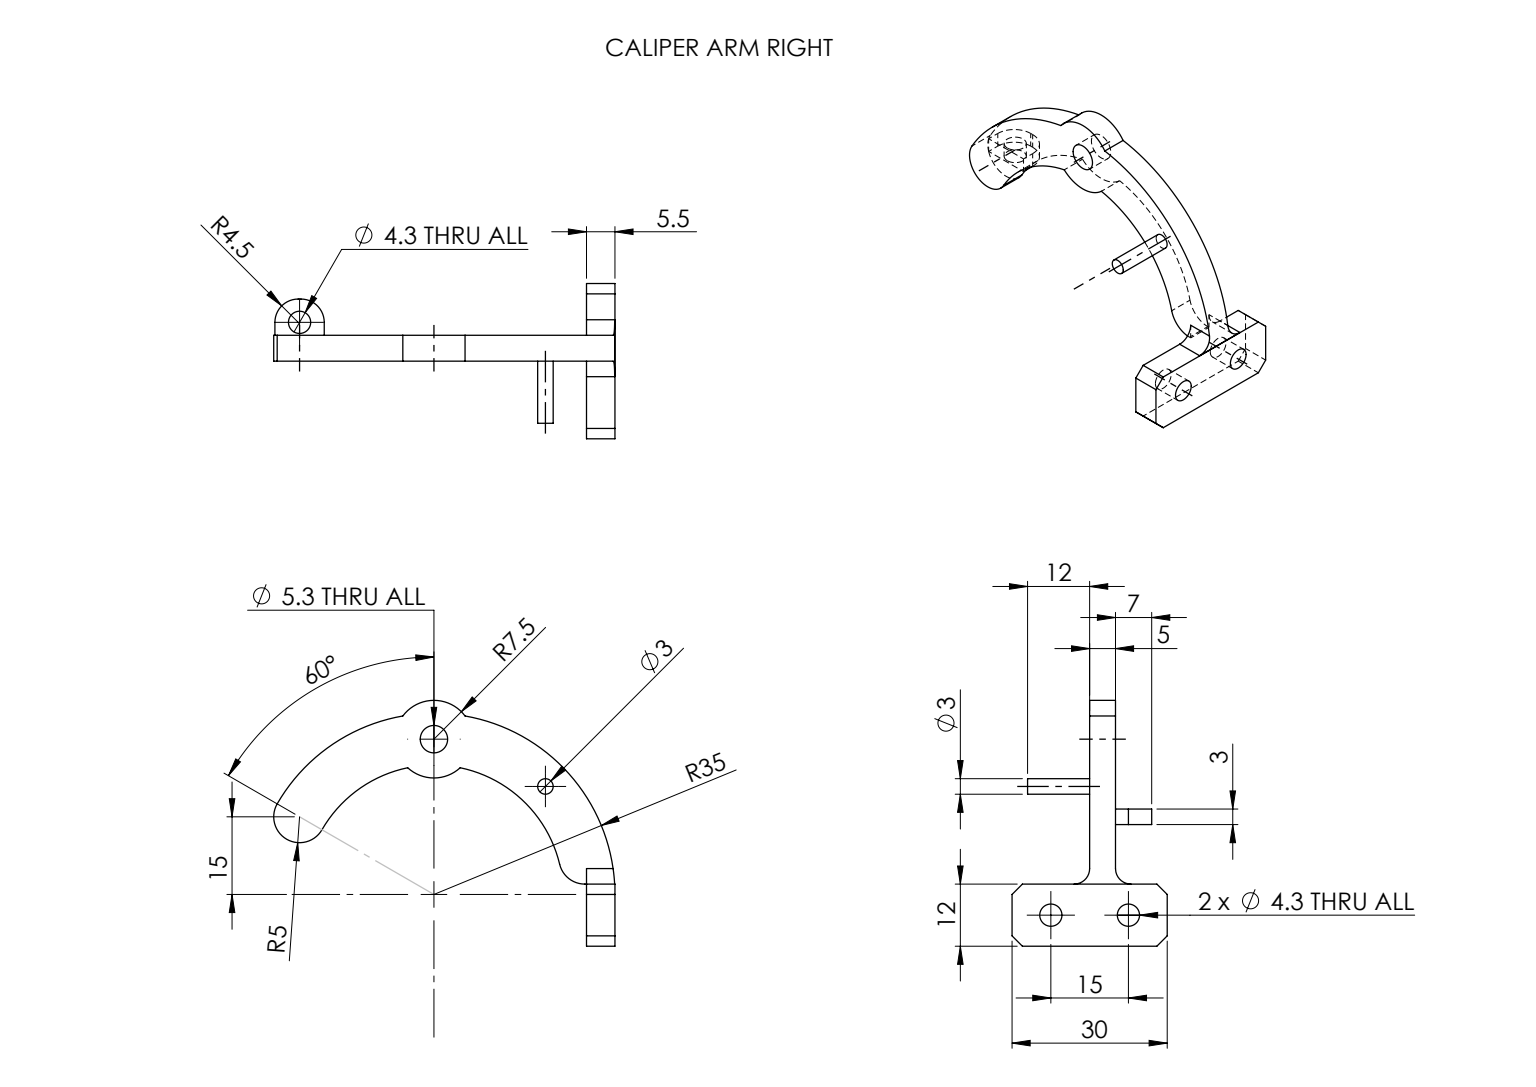
ISO-10303-21;
HEADER;
FILE_DESCRIPTION (('STEP AP214'),
    '1' );
FILE_NAME ('caliper arm right.step',
    '2026-10-08T05:45:04',
    ( '' ),
    ( '' ),
    'SwSTEP 2.0',
    'SolidWorks 2026',
    '' );
FILE_SCHEMA (( 'AUTOMOTIVE_DESIGN' ));
ENDSEC;

DATA;
#18=UNCERTAINTY_MEASURE_WITH_UNIT (LENGTH_MEASURE( 1.000000000000000082E-05 ), #5479, 'distance_accuracy_value', 'NONE');
#20=EDGE_CURVE ( 'NONE', #10326, #5059, #2301, .T. ) ;
#29=DIRECTION ( 'NONE',  ( 6.098637220230963674E-17, -1.000000000000000000, 0.000000000000000000 ) ) ;
#33=ADVANCED_FACE ( 'NONE', ( #727 ), #6680, .T. ) ;
#37=ORIENTED_EDGE ( 'NONE', *, *, #2342, .T. ) ;
#39=CARTESIAN_POINT ( 'NONE',  ( 34.64101615137754209, 5.000000000000000888, 2.500000000000000000 ) ) ;
#46=CARTESIAN_POINT ( 'NONE',  ( 29.49999999999999289, -3.999999999999993339, 12.14999999999999503 ) ) ;
#49=ADVANCED_FACE ( 'NONE', ( #5029 ), #6019, .T. ) ;
#84=LINE ( 'NONE', #3373, #8593 ) ;
#89=DIRECTION ( 'NONE',  ( 1.156482317317871478E-16, -0.000000000000000000, -1.000000000000000000 ) ) ;
#107=EDGE_CURVE ( 'NONE', #8667, #6915, #8632, .T. ) ;
#117=ORIENTED_EDGE ( 'NONE', *, *, #2558, .T. ) ;
#119=FILL_AREA_STYLE_COLOUR ( '', #3145 ) ;
#126=DIRECTION ( 'NONE',  ( -4.029251166000348040E-16, -0.7071067811865463515, 0.7071067811865486830 ) ) ;
#129=EDGE_CURVE ( 'NONE', #9236, #8327, #4531, .T. ) ;
#132=CARTESIAN_POINT ( 'NONE',  ( -30.75045812061784289, 13.49999999999941913, -5.000000000000000000 ) ) ;
#143=VERTEX_POINT ( 'NONE', #4423 ) ;
#157=DIRECTION ( 'NONE',  ( -1.000000000000000000, 0.000000000000000000, 0.000000000000000000 ) ) ;
#162=CARTESIAN_POINT ( 'NONE',  ( -6.015568632492056977, 34.47916666666665009, 0.000000000000000000 ) ) ;
#167=ADVANCED_FACE ( 'NONE', ( #9404 ), #2582, .F. ) ;
#169=DIRECTION ( 'NONE',  ( -1.000000000000000000, 0.000000000000000000, 0.000000000000000000 ) ) ;
#180=CARTESIAN_POINT ( 'NONE',  ( 0.000000000000000000, 0.000000000000000000, -2.500000000000000000 ) ) ;
#188=DIRECTION ( 'NONE',  ( 1.000000000000000000, 6.098637220230964906E-17, 0.000000000000000000 ) ) ;
#191=LINE ( 'NONE', #5261, #9329 ) ;
#195=CIRCLE ( 'NONE', #3924, 7.500000000000000000 ) ;
#203=EDGE_LOOP ( 'NONE', ( #3359, #5772 ) ) ;
#204=ORIENTED_EDGE ( 'NONE', *, *, #3358, .T. ) ;
#224=PRESENTATION_STYLE_ASSIGNMENT (( #9345 ) ) ;
#231=CARTESIAN_POINT ( 'NONE',  ( 34.99999999999999289, 2.000000000000002220, -12.49999999999999822 ) ) ;
#234=VERTEX_POINT ( 'NONE', #10467 ) ;
#236=EDGE_CURVE ( 'NONE', #3617, #2973, #5354, .T. ) ;
#238=DIRECTION ( 'NONE',  ( 0.000000000000000000, 0.000000000000000000, 1.000000000000000000 ) ) ;
#241=DIRECTION ( 'NONE',  ( 4.312387734421983755E-17, -0.7071067811865462405, -0.7071067811865489050 ) ) ;
#242=EDGE_CURVE ( 'NONE', #1228, #6486, #8792, .T. ) ;
#253=EDGE_CURVE ( 'NONE', #7504, #6853, #3627, .T. ) ;
#254=CARTESIAN_POINT ( 'NONE',  ( -25.98076211353324894, 16.50000000000026290, -7.149999999999990585 ) ) ;
#267=VECTOR ( 'NONE', #7158, 1000.000000000000000 ) ;
#268=DIRECTION ( 'NONE',  ( 0.000000000000000000, 0.000000000000000000, 1.000000000000000000 ) ) ;
#269=VECTOR ( 'NONE', #6345, 1000.000000000000000 ) ;
#270=VECTOR ( 'NONE', #9575, 1000.000000000000000 ) ;
#286=AXIS2_PLACEMENT_3D ( 'NONE', #4193, #3362, #6741 ) ;
#308=AXIS2_PLACEMENT_3D ( 'NONE', #6956, #4296, #9565 ) ;
#317=EDGE_LOOP ( 'NONE', ( #5235, #5389 ) ) ;
#326=CIRCLE ( 'NONE', #6705, 2.649999999999991029 ) ;
#331=CARTESIAN_POINT ( 'NONE',  ( -21.21106610644865498, 16.50000000000026290, -9.500000000000000000 ) ) ;
#334=ORIENTED_EDGE ( 'NONE', *, *, #9479, .T. ) ;
#342=ORIENTED_EDGE ( 'NONE', *, *, #1250, .F. ) ;
#346=CARTESIAN_POINT ( 'NONE',  ( -25.98076211353324894, 14.99999999999984190, -2.500000000000000000 ) ) ;
#348=CARTESIAN_POINT ( 'NONE',  ( -21.21106610644865498, 13.49999999999941913, -5.000000000000000000 ) ) ;
#350=CARTESIAN_POINT ( 'NONE',  ( 20.05579831881754060, 20.86490736922957367, 14.50000000000000000 ) ) ;
#360=ADVANCED_FACE ( 'NONE', ( #8018 ), #2971, .F. ) ;
#361=CARTESIAN_POINT ( 'NONE',  ( 34.99999999999999289, -3.999999999999993339, 10.00000000000000533 ) ) ;
#364=DIRECTION ( 'NONE',  ( 6.098637220230964906E-17, -1.000000000000000000, 0.000000000000000000 ) ) ;
#374=CYLINDRICAL_SURFACE ( 'NONE', #7364, 7.500000000000000000 ) ;
#398=DIRECTION ( 'NONE',  ( -4.312387734421998546E-17, 0.7071067811865489050, -0.7071067811865462405 ) ) ;
#420=VECTOR ( 'NONE', #4987, 1000.000000000000000 ) ;
#421=EDGE_CURVE ( 'NONE', #10496, #6333, #10386, .T. ) ;
#429=EDGE_CURVE ( 'NONE', #7102, #2953, #8173, .T. ) ;
#446=AXIS2_PLACEMENT_3D ( 'NONE', #473, #2203, #364 ) ;
#447=DIRECTION ( 'NONE',  ( 0.000000000000000000, 0.000000000000000000, -1.000000000000000000 ) ) ;
#448=FACE_BOUND ( 'NONE', #1109, .T. ) ;
#450=ORIENTED_EDGE ( 'NONE', *, *, #5486, .T. ) ;
#457=EDGE_CURVE ( 'NONE', #3885, #9988, #8075, .T. ) ;
#468=CARTESIAN_POINT ( 'NONE',  ( -25.71106610644865498, 13.49999999999941913, -5.000000000000000000 ) ) ;
#473=CARTESIAN_POINT ( 'NONE',  ( -3.049318610115482207E-16, 5.000000000000000000, -5.500000000000000000 ) ) ;
#480=DIRECTION ( 'NONE',  ( 0.000000000000000000, 0.000000000000000000, 1.000000000000000000 ) ) ;
#495=ORIENTED_EDGE ( 'NONE', *, *, #3771, .F. ) ;
#510=DIRECTION ( 'NONE',  ( 1.000000000000000000, 0.000000000000000000, 0.000000000000000000 ) ) ;
#515=UNCERTAINTY_MEASURE_WITH_UNIT (LENGTH_MEASURE( 1.000000000000000082E-05 ), #7040, 'distance_accuracy_value', 'NONE');
#517=DIRECTION ( 'NONE',  ( 0.000000000000000000, 0.000000000000000000, 1.000000000000000000 ) ) ;
#519=CARTESIAN_POINT ( 'NONE',  ( -25.98076211353324894, 13.49999999999941913, -7.149999999999990585 ) ) ;
#528=CARTESIAN_POINT ( 'NONE',  ( 0.000000000000000000, 0.000000000000000000, -2.500000000000000000 ) ) ;
#545=ADVANCED_FACE ( 'NONE', ( #10947 ), #7561, .T. ) ;
#551=ORIENTED_EDGE ( 'NONE', *, *, #3434, .F. ) ;
#555=EDGE_CURVE ( 'NONE', #6915, #590, #2328, .T. ) ;
#563=EDGE_LOOP ( 'NONE', ( #7565, #8832, #8917, #5557 ) ) ;
#564=DIRECTION ( 'NONE',  ( -1.000000000000000000, 0.000000000000000000, 0.000000000000000000 ) ) ;
#568=AXIS2_PLACEMENT_3D ( 'NONE', #528, #9502, #169 ) ;
#573=EDGE_CURVE ( 'NONE', #652, #6838, #3756, .T. ) ;
#575=FACE_OUTER_BOUND ( 'NONE', #2113, .T. ) ;
#577=ORIENTED_EDGE ( 'NONE', *, *, #9425, .T. ) ;
#589=ADVANCED_FACE ( 'NONE', ( #5232 ), #5948, .F. ) ;
#590=VERTEX_POINT ( 'NONE', #5013 ) ;
#599=AXIS2_PLACEMENT_3D ( 'NONE', #2316, #6635, #3978 ) ;
#603=EDGE_CURVE ( 'NONE', #9227, #143, #8788, .T. ) ;
#609=VERTEX_POINT ( 'NONE', #8450 ) ;
#616=DIRECTION ( 'NONE',  ( 1.000000000000000000, -0.000000000000000000, -0.000000000000000000 ) ) ;
#618=CARTESIAN_POINT ( 'NONE',  ( 34.99999999999999289, 2.000000000000002220, 15.50000000000000533 ) ) ;
#622=DIRECTION ( 'NONE',  ( -6.098637220230964906E-17, 1.000000000000000000, 0.000000000000000000 ) ) ;
#624=EDGE_CURVE ( 'NONE', #7008, #1215, #7866, .T. ) ;
#628=AXIS2_PLACEMENT_3D ( 'NONE', #1690, #8407, #6856 ) ;
#631=CARTESIAN_POINT ( 'NONE',  ( 29.49999999999999289, 2.000000000000001776, 17.50000000000000000 ) ) ;
#652=VERTEX_POINT ( 'NONE', #7794 ) ;
#659=CARTESIAN_POINT ( 'NONE',  ( 0.000000000000000000, 30.00000000000000000, -2.499999999999998668 ) ) ;
#663=AXIS2_PLACEMENT_3D ( 'NONE', #9560, #2957, #1054 ) ;
#666=PRODUCT_DEFINITION_CONTEXT ( 'detailed design', #7209, 'design' ) ;
#667=ORIENTED_EDGE ( 'NONE', *, *, #6516, .T. ) ;
#670=VERTEX_POINT ( 'NONE', #1318 ) ;
#672=VECTOR ( 'NONE', #10406, 1000.000000000000000 ) ;
#674=VECTOR ( 'NONE', #5477, 1000.000000000000000 ) ;
#680=DIRECTION ( 'NONE',  ( -0.000000000000000000, -0.000000000000000000, -1.000000000000000000 ) ) ;
#690=EDGE_LOOP ( 'NONE', ( #9028, #6042, #6525, #4019, #7005, #10810 ) ) ;
#691=DIRECTION ( 'NONE',  ( -1.000000000000000000, -6.098637220230964906E-17, -0.000000000000000000 ) ) ;
#727=FACE_OUTER_BOUND ( 'NONE', #7562, .T. ) ;
#730=EDGE_LOOP ( 'NONE', ( #3773, #3925, #4540, #10930 ) ) ;
#752=DIRECTION ( 'NONE',  ( 1.000000000000000000, -0.000000000000000000, -0.000000000000000000 ) ) ;
#753=EDGE_LOOP ( 'NONE', ( #8453, #4556, #9444, #8263 ) ) ;
#761=EDGE_CURVE ( 'NONE', #652, #9304, #1958, .T. ) ;
#763=LINE ( 'NONE', #4112, #7788 ) ;
#768=ORIENTED_EDGE ( 'NONE', *, *, #5709, .F. ) ;
#777=LINE ( 'NONE', #3237, #3403 ) ;
#780=AXIS2_PLACEMENT_3D ( 'NONE', #1700, #10147, #4202 ) ;
#785=PLANE ( 'NONE',  #286 ) ;
#793=EDGE_CURVE ( 'NONE', #10021, #7800, #2005, .T. ) ;
#798=VECTOR ( 'NONE', #7045, 1000.000000000000000 ) ;
#803=CARTESIAN_POINT ( 'NONE',  ( -5.076455387921338769, 24.47916666666667140, 0.000000000000000000 ) ) ;
#809=ORIENTED_EDGE ( 'NONE', *, *, #7983, .T. ) ;
#811=ORIENTED_EDGE ( 'NONE', *, *, #6656, .T. ) ;
#812=CARTESIAN_POINT ( 'NONE',  ( 29.49999999999999289, 2.000000000000001776, 2.500000000000000000 ) ) ;
#814=CARTESIAN_POINT ( 'NONE',  ( 29.49999999999999289, 5.000000000000000888, 2.500000000000000000 ) ) ;
#816=ORIENTED_EDGE ( 'NONE', *, *, #6670, .T. ) ;
#820=CARTESIAN_POINT ( 'NONE',  ( -25.71106610644865498, 0.000000000000000000, -9.500000000000000000 ) ) ;
#828=DIRECTION ( 'NONE',  ( -1.000000000000000000, 0.000000000000000000, 0.000000000000000000 ) ) ;
#833=CIRCLE ( 'NONE', #5635, 24.99999999999999645 ) ;
#836=ORIENTED_EDGE ( 'NONE', *, *, #9189, .T. ) ;
#838=EDGE_CURVE ( 'NONE', #2609, #10326, #4874, .T. ) ;
#862=DIRECTION ( 'NONE',  ( -1.000000000000000000, 0.000000000000000000, 0.000000000000000000 ) ) ;
#863=ORIENTED_EDGE ( 'NONE', *, *, #7983, .F. ) ;
#865=CARTESIAN_POINT ( 'NONE',  ( -30.75045812061784289, 16.50000000000026290, -2.500000000000000000 ) ) ;
#873=DIRECTION ( 'NONE',  ( -0.000000000000000000, 1.000000000000000000, 0.000000000000000000 ) ) ;
#877=EDGE_LOOP ( 'NONE', ( #6365, #5510 ) ) ;
#879=CARTESIAN_POINT ( 'NONE',  ( 29.49999999999999645, -7.999999999999996447, -12.49999999999999822 ) ) ;
#887=ORIENTED_EDGE ( 'NONE', *, *, #8923, .F. ) ;
#906=DIRECTION ( 'NONE',  ( -1.000000000000000000, 0.000000000000000000, 0.000000000000000000 ) ) ;
#908=CARTESIAN_POINT ( 'NONE',  ( 34.94281041931228771, 2.000000000000002220, -5.301324476612965242 ) ) ;
#910=PLANE ( 'NONE',  #3395 ) ;
#929=DIRECTION ( 'NONE',  ( -0.000000000000000000, 0.000000000000000000, -1.000000000000000000 ) ) ;
#942=DIRECTION ( 'NONE',  ( 0.000000000000000000, 0.000000000000000000, 1.000000000000000000 ) ) ;
#949=SHAPE_REPRESENTATION_RELATIONSHIP ( 'NONE' , 'NONE' ,  #10603, #6795 ) ;
#954=DIRECTION ( 'NONE',  ( 0.000000000000000000, 1.000000000000000000, 0.000000000000000000 ) ) ;
#959=AXIS2_PLACEMENT_3D ( 'NONE', #6647, #5113, #988 ) ;
#970=DIRECTION ( 'NONE',  ( 0.000000000000000000, 1.000000000000000000, 0.000000000000000000 ) ) ;
#984=FACE_OUTER_BOUND ( 'NONE', #2842, .T. ) ;
#988=DIRECTION ( 'NONE',  ( 0.000000000000000000, 1.000000000000000000, 0.000000000000000000 ) ) ;
#1001=EDGE_LOOP ( 'NONE', ( #342, #7622, #3380, #7323 ) ) ;
#1010=VECTOR ( 'NONE', #8855, 1000.000000000000000 ) ;
#1019=CIRCLE ( 'NONE', #10430, 2.149999999999992362 ) ;
#1040=ORIENTED_EDGE ( 'NONE', *, *, #5486, .F. ) ;
#1046=FACE_OUTER_BOUND ( 'NONE', #9517, .T. ) ;
#1054=DIRECTION ( 'NONE',  ( -1.000000000000000000, 0.000000000000000000, 0.000000000000000000 ) ) ;
#1059=EDGE_CURVE ( 'NONE', #10287, #9304, #1463, .T. ) ;
#1066=ORIENTED_EDGE ( 'NONE', *, *, #8871, .F. ) ;
#1067=ORIENTED_EDGE ( 'NONE', *, *, #9101, .F. ) ;
#1074=CARTESIAN_POINT ( 'NONE',  ( -21.21106610644865498, 13.49999999999941913, -2.500000000000000000 ) ) ;
#1075=PLANE ( 'NONE',  #2989 ) ;
#1078=CYLINDRICAL_SURFACE ( 'NONE', #1884, 4.500000000000000000 ) ;
#1091=ORIENTED_EDGE ( 'NONE', *, *, #8045, .T. ) ;
#1109=EDGE_LOOP ( 'NONE', ( #1439, #1605 ) ) ;
#1112=ORIENTED_EDGE ( 'NONE', *, *, #5214, .F. ) ;
#1117=EDGE_CURVE ( 'NONE', #4463, #7719, #5019, .T. ) ;
#1147=AXIS2_PLACEMENT_3D ( 'NONE', #7692, #126, #9234 ) ;
#1151=CARTESIAN_POINT ( 'NONE',  ( 29.17190429162963738, 6.999999999999999112, 2.500000000000000000 ) ) ;
#1158=VECTOR ( 'NONE', #7928, 1000.000000000000000 ) ;
#1173=CIRCLE ( 'NONE', #2600, 4.999999999999997335 ) ;
#1189=FACE_BOUND ( 'NONE', #5424, .T. ) ;
#1201=CARTESIAN_POINT ( 'NONE',  ( 23.05579831881754416, 20.86490736922957367, 14.50000000000000000 ) ) ;
#1210=ORIENTED_EDGE ( 'NONE', *, *, #6774, .F. ) ;
#1215=VERTEX_POINT ( 'NONE', #5273 ) ;
#1220=DIRECTION ( 'NONE',  ( 0.000000000000000000, 0.000000000000000000, 1.000000000000000000 ) ) ;
#1226=ORIENTED_EDGE ( 'NONE', *, *, #5735, .F. ) ;
#1228=VERTEX_POINT ( 'NONE', #4446 ) ;
#1236=CARTESIAN_POINT ( 'NONE',  ( -21.21106610644865498, 13.49999999999941913, -2.500000000000000000 ) ) ;
#1246=CARTESIAN_POINT ( 'NONE',  ( 0.000000000000000000, 0.000000000000000000, 2.500000000000000000 ) ) ;
#1247=DIRECTION ( 'NONE',  ( 0.000000000000000000, 0.000000000000000000, 1.000000000000000000 ) ) ;
#1250=EDGE_CURVE ( 'NONE', #6186, #3385, #6758, .T. ) ;
#1255=FACE_BOUND ( 'NONE', #7518, .T. ) ;
#1263=CARTESIAN_POINT ( 'NONE',  ( 29.49999999999999645, 2.000000000000001776, -12.49999999999999822 ) ) ;
#1271=EDGE_CURVE ( 'NONE', #6186, #3429, #7100, .T. ) ;
#1277=CARTESIAN_POINT ( 'NONE',  ( 29.49999999999999645, 2.000000000000001776, -12.49999999999999822 ) ) ;
#1280=LINE ( 'NONE', #3985, #5818 ) ;
#1283=ORIENTED_EDGE ( 'NONE', *, *, #6189, .T. ) ;
#1294=DIRECTION ( 'NONE',  ( -0.000000000000000000, -0.000000000000000000, 1.000000000000000000 ) ) ;
#1300=CARTESIAN_POINT ( 'NONE',  ( 34.94281041931228771, 2.000000000000002220, 5.500000000000000000 ) ) ;
#1317=ORIENTED_EDGE ( 'NONE', *, *, #7967, .T. ) ;
#1318=CARTESIAN_POINT ( 'NONE',  ( 24.30992024302469900, 5.833333333333329485, 2.500000000000000000 ) ) ;
#1329=AXIS2_PLACEMENT_3D ( 'NONE', #7945, #2115, #8886 ) ;
#1331=CARTESIAN_POINT ( 'NONE',  ( -5.076455387921339657, 24.47916666666667140, -2.499999999999998668 ) ) ;
#1342=AXIS2_PLACEMENT_3D ( 'NONE', #10221, #4336, #7725 ) ;
#1351=VERTEX_POINT ( 'NONE', #3601 ) ;
#1359=DIRECTION ( 'NONE',  ( 1.000000000000000000, 6.098637220230964906E-17, 0.000000000000000000 ) ) ;
#1361=CARTESIAN_POINT ( 'NONE',  ( 23.05579831881754416, 20.86490736922957367, 2.500000000000000444 ) ) ;
#1362=VERTEX_POINT ( 'NONE', #3710 ) ;
#1372=CARTESIAN_POINT ( 'NONE',  ( -26.25045812061784289, 16.50000000000026290, -5.000000000000000000 ) ) ;
#1381=ORIENTED_EDGE ( 'NONE', *, *, #2352, .F. ) ;
#1386=VERTEX_POINT ( 'NONE', #2997 ) ;
#1389=CARTESIAN_POINT ( 'NONE',  ( 34.94281041931228771, 2.000000000000002220, 5.500000000000000000 ) ) ;
#1433=EDGE_CURVE ( 'NONE', #7860, #7488, #1942, .T. ) ;
#1438=DIRECTION ( 'NONE',  ( -0.000000000000000000, -0.000000000000000000, -1.000000000000000000 ) ) ;
#1439=ORIENTED_EDGE ( 'NONE', *, *, #8318, .F. ) ;
#1452=DIRECTION ( 'NONE',  ( -0.000000000000000000, -0.000000000000000000, -1.000000000000000000 ) ) ;
#1459=EDGE_CURVE ( 'NONE', #7662, #1215, #7307, .T. ) ;
#1463=CIRCLE ( 'NONE', #2896, 2.149999999999992362 ) ;
#1474=CARTESIAN_POINT ( 'NONE',  ( 21.55579831881754416, 20.86490736922957367, 14.50000000000000000 ) ) ;
#1488=AXIS2_PLACEMENT_3D ( 'NONE', #9432, #873, #7663 ) ;
#1491=VERTEX_POINT ( 'NONE', #6470 ) ;
#1507=VECTOR ( 'NONE', #9328, 1000.000000000000114 ) ;
#1513=AXIS2_PLACEMENT_3D ( 'NONE', #3252, #4934, #862 ) ;
#1520=ADVANCED_FACE ( 'NONE', ( #575 ), #4820, .F. ) ;
#1528=DIRECTION ( 'NONE',  ( 4.312387734421982522E-17, -0.7071067811865462405, 0.7071067811865489050 ) ) ;
#1529=FACE_OUTER_BOUND ( 'NONE', #4996, .T. ) ;
#1544=ORIENTED_EDGE ( 'NONE', *, *, #1599, .F. ) ;
#1545=ORIENTED_EDGE ( 'NONE', *, *, #7499, .T. ) ;
#1549=CARTESIAN_POINT ( 'NONE',  ( -30.31088913245546124, 17.49999999999980815, 2.500000000000000000 ) ) ;
#1551=ORIENTED_EDGE ( 'NONE', *, *, #2352, .T. ) ;
#1552=CIRCLE ( 'NONE', #7059, 2.149999999999990585 ) ;
#1560=CARTESIAN_POINT ( 'NONE',  ( 25.58039891549807976, 2.000000000000001776, 2.500000000000000000 ) ) ;
#1568=VECTOR ( 'NONE', #954, 1000.000000000000000 ) ;
#1580=CARTESIAN_POINT ( 'NONE',  ( 29.17190429162964094, 2.000000000000001776, -2.500000000000000444 ) ) ;
#1582=DIRECTION ( 'NONE',  ( -0.000000000000000000, -0.000000000000000000, -1.000000000000000000 ) ) ;
#1594=EDGE_CURVE ( 'NONE', #2434, #1351, #2285, .T. ) ;
#1599=EDGE_CURVE ( 'NONE', #6333, #10496, #326, .T. ) ;
#1605=ORIENTED_EDGE ( 'NONE', *, *, #8341, .F. ) ;
#1613=DIRECTION ( 'NONE',  ( 0.000000000000000000, -0.000000000000000000, 1.000000000000000000 ) ) ;
#1615=AXIS2_PLACEMENT_3D ( 'NONE', #1474, #6623, #6692 ) ;
#1616=CARTESIAN_POINT ( 'NONE',  ( 29.49999999999999289, -3.999999999999993339, 10.00000000000000533 ) ) ;
#1622=EDGE_CURVE ( 'NONE', #2973, #8252, #3368, .T. ) ;
#1631=CARTESIAN_POINT ( 'NONE',  ( 29.49999999999999289, 6.938893903907228378E-15, 17.50000000000000000 ) ) ;
#1636=FACE_OUTER_BOUND ( 'NONE', #10823, .T. ) ;
#1638=LINE ( 'NONE', #5034, #10552 ) ;
#1643=CARTESIAN_POINT ( 'NONE',  ( 0.000000000000000000, 30.00000000000000000, 2.500000000000000000 ) ) ;
#1646=VECTOR ( 'NONE', #2791, 1000.000000000000000 ) ;
#1653=ORIENTED_EDGE ( 'NONE', *, *, #10884, .F. ) ;
#1660=FACE_OUTER_BOUND ( 'NONE', #9991, .T. ) ;
#1670=DIRECTION ( 'NONE',  ( -1.000000000000000000, -6.098637220230963674E-17, -1.156482317317871725E-16 ) ) ;
#1671=ORIENTED_EDGE ( 'NONE', *, *, #9189, .F. ) ;
#1684=PLANE ( 'NONE',  #1709 ) ;
#1687=VERTEX_POINT ( 'NONE', #5154 ) ;
#1690=CARTESIAN_POINT ( 'NONE',  ( -25.71106610644865498, 16.50000000000026290, -5.000000000000000000 ) ) ;
#1691=VECTOR ( 'NONE', #89, 1000.000000000000000 ) ;
#1700=CARTESIAN_POINT ( 'NONE',  ( 0.000000000000000000, 0.000000000000000000, 2.500000000000000000 ) ) ;
#1701=CARTESIAN_POINT ( 'NONE',  ( 0.000000000000000000, 0.000000000000000000, 2.500000000000000000 ) ) ;
#1709=AXIS2_PLACEMENT_3D ( 'NONE', #1631, #10902, #8291 ) ;
#1710=DIRECTION ( 'NONE',  ( 0.000000000000000000, 0.000000000000000000, -1.000000000000000000 ) ) ;
#1716=FACE_OUTER_BOUND ( 'NONE', #7064, .T. ) ;
#1721=CARTESIAN_POINT ( 'NONE',  ( 0.000000000000000000, 30.00000000000000000, -2.500000000000000000 ) ) ;
#1729=EDGE_CURVE ( 'NONE', #590, #6915, #9910, .T. ) ;
#1731=DIRECTION ( 'NONE',  ( -1.000000000000000000, -6.098637220230963674E-17, -1.156482317317871725E-16 ) ) ;
#1733=LINE ( 'NONE', #10949, #4942 ) ;
#1789=DIRECTION ( 'NONE',  ( 0.000000000000000000, 0.000000000000000000, 1.000000000000000000 ) ) ;
#1790=ORIENTED_EDGE ( 'NONE', *, *, #7191, .F. ) ;
#1791=DIRECTION ( 'NONE',  ( 4.312387734421997313E-17, -0.7071067811865486830, -0.7071067811865463515 ) ) ;
#1804=VERTEX_POINT ( 'NONE', #6362 ) ;
#1821=CARTESIAN_POINT ( 'NONE',  ( 29.49999999999999645, 2.000000000000001776, -12.49999999999999822 ) ) ;
#1856=VECTOR ( 'NONE', #29, 1000.000000000000000 ) ;
#1857=LINE ( 'NONE', #132, #6662 ) ;
#1862=LINE ( 'NONE', #7700, #3214 ) ;
#1865=ADVANCED_FACE ( 'NONE', ( #1189, #7978 ), #2090, .F. ) ;
#1882=CARTESIAN_POINT ( 'NONE',  ( 34.99999999999999289, 2.000000000000002220, 17.50000000000000355 ) ) ;
#1884=AXIS2_PLACEMENT_3D ( 'NONE', #10480, #970, #6865 ) ;
#1898=EDGE_CURVE ( 'NONE', #8716, #10904, #763, .T. ) ;
#1903=CARTESIAN_POINT ( 'NONE',  ( -2.649999999999991029, 30.00000000000000000, -2.500000000000000000 ) ) ;
#1916=DIRECTION ( 'NONE',  ( -1.000000000000000000, 0.000000000000000000, 0.000000000000000000 ) ) ;
#1923=PLANE ( 'NONE',  #7910 ) ;
#1930=CARTESIAN_POINT ( 'NONE',  ( -21.21106610644865498, 16.50000000000026290, -2.500000000000000000 ) ) ;
#1932=SURFACE_SIDE_STYLE ('',( #9148 ) ) ;
#1939=LINE ( 'NONE', #254, #798 ) ;
#1942=LINE ( 'NONE', #6205, #9085 ) ;
#1948=ADVANCED_FACE ( 'NONE', ( #10944 ), #6723, .T. ) ;
#1949=LINE ( 'NONE', #7154, #8068 ) ;
#1958=LINE ( 'NONE', #7002, #1646 ) ;
#1971=EDGE_LOOP ( 'NONE', ( #9546, #6752, #9684, #9152 ) ) ;
#1977=DIRECTION ( 'NONE',  ( 0.000000000000000000, 0.000000000000000000, -1.000000000000000000 ) ) ;
#1978=LINE ( 'NONE', #350, #9543 ) ;
#1982=CARTESIAN_POINT ( 'NONE',  ( -25.98076211353324894, 13.49999999999941913, -5.000000000000000000 ) ) ;
#1995=DIRECTION ( 'NONE',  ( 1.000000000000000000, 6.098637220230964906E-17, 0.000000000000000000 ) ) ;
#2005=LINE ( 'NONE', #2364, #10865 ) ;
#2022=CARTESIAN_POINT ( 'NONE',  ( -21.65063509461104374, 12.49999999999986322, -2.500000000000000000 ) ) ;
#2030=CIRCLE ( 'NONE', #10190, 5.000000000000000888 ) ;
#2038=CARTESIAN_POINT ( 'NONE',  ( 29.49999999999999289, -7.999999999999996447, 17.50000000000000000 ) ) ;
#2044=CIRCLE ( 'NONE', #5244, 4.999999999999997335 ) ;
#2046=VECTOR ( 'NONE', #6825, 1000.000000000000000 ) ;
#2048=DIRECTION ( 'NONE',  ( 0.000000000000000000, 0.000000000000000000, 1.000000000000000000 ) ) ;
#2049=CARTESIAN_POINT ( 'NONE',  ( 34.94281041931228771, 2.000000000000002220, -5.500000000000000000 ) ) ;
#2053=VECTOR ( 'NONE', #9065, 1000.000000000000000 ) ;
#2069=DIRECTION ( 'NONE',  ( 0.000000000000000000, 0.000000000000000000, -1.000000000000000000 ) ) ;
#2070=ADVANCED_FACE ( 'NONE', ( #4696 ), #6294, .T. ) ;
#2076=CARTESIAN_POINT ( 'NONE',  ( 2.649999999999991029, 30.00000000000000000, -2.500000000000000000 ) ) ;
#2077=ORIENTED_EDGE ( 'NONE', *, *, #6021, .F. ) ;
#2087=CARTESIAN_POINT ( 'NONE',  ( 29.17190429162963738, 6.999999999999999112, -2.500000000000000000 ) ) ;
#2090=PLANE ( 'NONE',  #3345 ) ;
#2095=AXIS2_PLACEMENT_3D ( 'NONE', #2695, #7635, #1916 ) ;
#2107=ORIENTED_EDGE ( 'NONE', *, *, #6968, .F. ) ;
#2112=SHAPE_DEFINITION_REPRESENTATION ( #2630, #10603 ) ;
#2113=EDGE_LOOP ( 'NONE', ( #6669, #9050, #7283, #4140 ) ) ;
#2115=DIRECTION ( 'NONE',  ( -0.000000000000000000, 1.000000000000000000, -0.000000000000000000 ) ) ;
#2117=AXIS2_PLACEMENT_3D ( 'NONE', #8865, #1247, #510 ) ;
#2123=ORIENTED_EDGE ( 'NONE', *, *, #242, .T. ) ;
#2132=DIRECTION ( 'NONE',  ( 0.000000000000000000, 0.000000000000000000, 1.000000000000000000 ) ) ;
#2134=VERTEX_POINT ( 'NONE', #10528 ) ;
#2147=EDGE_CURVE ( 'NONE', #7593, #609, #6240, .T. ) ;
#2156=VECTOR ( 'NONE', #5024, 1000.000000000000000 ) ;
#2167=EDGE_CURVE ( 'NONE', #7719, #4463, #2464, .T. ) ;
#2192=DIRECTION ( 'NONE',  ( 1.000000000000000000, 6.098637220230963674E-17, -0.000000000000000000 ) ) ;
#2201=EDGE_CURVE ( 'NONE', #9227, #3885, #4970, .T. ) ;
#2203=DIRECTION ( 'NONE',  ( -1.000000000000000000, -6.098637220230964906E-17, 0.000000000000000000 ) ) ;
#2243=DIRECTION ( 'NONE',  ( 0.000000000000000000, 0.000000000000000000, -1.000000000000000000 ) ) ;
#2253=CARTESIAN_POINT ( 'NONE',  ( 29.49999999999999289, -3.999999999999993339, 10.00000000000000533 ) ) ;
#2271=AXIS2_PLACEMENT_3D ( 'NONE', #8903, #3738, #2132 ) ;
#2275=CARTESIAN_POINT ( 'NONE',  ( 34.92403196580097813, 2.306010598194980332, 4.165547504151214220 ) ) ;
#2277=ORIENTED_EDGE ( 'NONE', *, *, #1271, .F. ) ;
#2278=FACE_BOUND ( 'NONE', #9260, .T. ) ;
#2281=MECHANICAL_DESIGN_GEOMETRIC_PRESENTATION_REPRESENTATION('',(#9019),#3880);
#2284=ORIENTED_EDGE ( 'NONE', *, *, #129, .T. ) ;
#2285=CIRCLE ( 'NONE', #5820, 4.500000000000000000 ) ;
#2298=LINE ( 'NONE', #8228, #3052 ) ;
#2301=LINE ( 'NONE', #7460, #8418 ) ;
#2302=DIRECTION ( 'NONE',  ( 0.000000000000000000, 0.000000000000000000, 1.000000000000000000 ) ) ;
#2303=ORIENTED_EDGE ( 'NONE', *, *, #1059, .T. ) ;
#2316=CARTESIAN_POINT ( 'NONE',  ( -26.25045812061784289, 13.49999999999941913, -5.000000000000000000 ) ) ;
#2320=EDGE_LOOP ( 'NONE', ( #5295, #8237 ) ) ;
#2322=ORIENTED_EDGE ( 'NONE', *, *, #6099, .F. ) ;
#2325=ORIENTED_EDGE ( 'NONE', *, *, #107, .T. ) ;
#2328=CIRCLE ( 'NONE', #9427, 2.149999999999992362 ) ;
#2342=EDGE_CURVE ( 'NONE', #1362, #1687, #195, .T. ) ;
#2352=EDGE_CURVE ( 'NONE', #5059, #3529, #8459, .T. ) ;
#2364=CARTESIAN_POINT ( 'NONE',  ( -1.219727444046192735E-16, 2.000000000000000000, 5.500000000000000000 ) ) ;
#2372=ORIENTED_EDGE ( 'NONE', *, *, #10918, .T. ) ;
#2374=EDGE_LOOP ( 'NONE', ( #4836, #3850, #10797, #816, #117, #3301, #37, #1091, #9343, #10366, #204, #10004 ) ) ;
#2384=VECTOR ( 'NONE', #9155, 1000.000000000000000 ) ;
#2390=LINE ( 'NONE', #9224, #4040 ) ;
#2395=ORIENTED_EDGE ( 'NONE', *, *, #10128, .T. ) ;
#2402=CIRCLE ( 'NONE', #10922, 24.99999999999999645 ) ;
#2407=CYLINDRICAL_SURFACE ( 'NONE', #9005, 4.999999999999997335 ) ;
#2408=ORIENTED_EDGE ( 'NONE', *, *, #4921, .T. ) ;
#2416=LINE ( 'NONE', #9811, #4894 ) ;
#2421=CARTESIAN_POINT ( 'NONE',  ( -21.21106610644865498, 13.49999999999941913, -9.500000000000000000 ) ) ;
#2423=ORIENTED_EDGE ( 'NONE', *, *, #8672, .T. ) ;
#2434=VERTEX_POINT ( 'NONE', #2478 ) ;
#2438=CARTESIAN_POINT ( 'NONE',  ( -6.015568632492068524, 34.47916666666665719, -2.499999999999998668 ) ) ;
#2439=EDGE_LOOP ( 'NONE', ( #4240, #4235, #811, #836 ) ) ;
#2447=DIRECTION ( 'NONE',  ( -1.000000000000000000, -2.775557561562891351E-15, 0.000000000000000000 ) ) ;
#2464=CIRCLE ( 'NONE', #2117, 1.500000000000001332 ) ;
#2465=CARTESIAN_POINT ( 'NONE',  ( 0.000000000000000000, 30.00000000000000000, 2.500000000000000000 ) ) ;
#2468=FACE_OUTER_BOUND ( 'NONE', #8896, .T. ) ;
#2470=PLANE ( 'NONE',  #4212 ) ;
#2472=ORIENTED_EDGE ( 'NONE', *, *, #5726, .T. ) ;
#2478=CARTESIAN_POINT ( 'NONE',  ( -26.25045812061784289, 16.50000000000026290, -9.500000000000000000 ) ) ;
#2482=CARTESIAN_POINT ( 'NONE',  ( 34.99999999999999289, -7.999999999999996447, 17.50000000000000355 ) ) ;
#2493=DIRECTION ( 'NONE',  ( -1.000000000000000000, 0.000000000000000000, 0.000000000000000000 ) ) ;
#2502=ADVANCED_FACE ( 'NONE', ( #1529 ), #3308, .T. ) ;
#2503=DIRECTION ( 'NONE',  ( -1.000000000000000000, 0.000000000000000000, 0.000000000000000000 ) ) ;
#2515=DIRECTION ( 'NONE',  ( -3.865177154555985764E-17, -0.7071067811865489050, 0.7071067811865462405 ) ) ;
#2518=DIRECTION ( 'NONE',  ( -1.000000000000000000, 0.000000000000000000, 0.000000000000000000 ) ) ;
#2525=CARTESIAN_POINT ( 'NONE',  ( 34.93373351399775117, 2.154066368359275785, -4.530732988813361395 ) ) ;
#2551=CARTESIAN_POINT ( 'NONE',  ( 0.000000000000000000, 30.00000000000000000, -2.500000000000000000 ) ) ;
#2554=LINE ( 'NONE', #5939, #1507 ) ;
#2558=EDGE_CURVE ( 'NONE', #7683, #6952, #1862, .T. ) ;
#2572=SURFACE_SIDE_STYLE ('',( #7742 ) ) ;
#2582=CYLINDRICAL_SURFACE ( 'NONE', #9851, 2.149999999999987921 ) ;
#2591=UNCERTAINTY_MEASURE_WITH_UNIT (LENGTH_MEASURE( 1.000000000000000082E-05 ), #2637, 'distance_accuracy_value', 'NONE');
#2600=AXIS2_PLACEMENT_3D ( 'NONE', #9069, #10796, #4973 ) ;
#2602=EDGE_CURVE ( 'NONE', #1804, #4007, #7123, .T. ) ;
#2607=CARTESIAN_POINT ( 'NONE',  ( 21.55579831881754416, 20.86490736922957367, 14.50000000000000000 ) ) ;
#2609=VERTEX_POINT ( 'NONE', #1074 ) ;
#2612=ADVANCED_FACE ( 'NONE', ( #6080, #2817 ), #910, .F. ) ;
#2625=EDGE_CURVE ( 'NONE', #5721, #2134, #3045, .T. ) ;
#2630=PRODUCT_DEFINITION_SHAPE ( 'NONE', 'NONE',  #2815 ) ;
#2631=ORIENTED_EDGE ( 'NONE', *, *, #5215, .F. ) ;
#2635=ORIENTED_EDGE ( 'NONE', *, *, #421, .T. ) ;
#2637=( LENGTH_UNIT ( ) NAMED_UNIT ( * ) SI_UNIT ( .MILLI., .METRE. ) );
#2639=CIRCLE ( 'NONE', #663, 1.500000000000001332 ) ;
#2652=CARTESIAN_POINT ( 'NONE',  ( 34.82492259089467979, 3.500278077966952228, -2.894288569839196690 ) ) ;
#2656=DIRECTION ( 'NONE',  ( 0.000000000000000000, 0.000000000000000000, 1.000000000000000000 ) ) ;
#2667=ORIENTED_EDGE ( 'NONE', *, *, #7486, .T. ) ;
#2695=CARTESIAN_POINT ( 'NONE',  ( -25.98076211353324894, 14.99999999999984190, 2.500000000000000000 ) ) ;
#2696=ORIENTED_EDGE ( 'NONE', *, *, #10557, .T. ) ;
#2737=ORIENTED_EDGE ( 'NONE', *, *, #429, .T. ) ;
#2738=EDGE_CURVE ( 'NONE', #1491, #1362, #4642, .T. ) ;
#2740=( NAMED_UNIT ( * ) SI_UNIT ( $, .STERADIAN. ) SOLID_ANGLE_UNIT ( ) );
#2746=DIRECTION ( 'NONE',  ( -1.000000000000000000, 0.000000000000000000, 0.000000000000000000 ) ) ;
#2757=DIRECTION ( 'NONE',  ( 1.000000000000000000, 6.098637220230963674E-17, 1.156482317317871725E-16 ) ) ;
#2761=LINE ( 'NONE', #8645, #3996 ) ;
#2784=DIRECTION ( 'NONE',  ( -0.000000000000000000, -0.000000000000000000, -1.000000000000000000 ) ) ;
#2785=AXIS2_PLACEMENT_3D ( 'NONE', #9408, #7812, #9519 ) ;
#2791=DIRECTION ( 'NONE',  ( 1.000000000000000000, -0.000000000000000000, -0.000000000000000000 ) ) ;
#2793=LINE ( 'NONE', #6222, #3521 ) ;
#2805=AXIS2_PLACEMENT_3D ( 'NONE', #3700, #2192, #8085 ) ;
#2809=ORIENTED_EDGE ( 'NONE', *, *, #129, .F. ) ;
#2812=LINE ( 'NONE', #6188, #270 ) ;
#2815=PRODUCT_DEFINITION ( 'UNKNOWN', '', #6336, #666 ) ;
#2817=FACE_OUTER_BOUND ( 'NONE', #4834, .T. ) ;
#2837=ORIENTED_EDGE ( 'NONE', *, *, #5493, .F. ) ;
#2842=EDGE_LOOP ( 'NONE', ( #10161, #8175, #2423, #2303 ) ) ;
#2845=DIRECTION ( 'NONE',  ( 1.000000000000000000, 0.000000000000000000, 0.000000000000000000 ) ) ;
#2856=EDGE_CURVE ( 'NONE', #143, #9988, #777, .T. ) ;
#2866=DIRECTION ( 'NONE',  ( -1.000000000000000000, 0.000000000000000000, 0.000000000000000000 ) ) ;
#2884=CYLINDRICAL_SURFACE ( 'NONE', #7299, 2.149999999999987921 ) ;
#2896=AXIS2_PLACEMENT_3D ( 'NONE', #5048, #6706, #1710 ) ;
#2900=EDGE_CURVE ( 'NONE', #8252, #8716, #2298, .T. ) ;
#2913=DIRECTION ( 'NONE',  ( 6.098637220230963674E-17, -1.000000000000000000, 0.000000000000000000 ) ) ;
#2937=DIRECTION ( 'NONE',  ( 0.000000000000000000, 0.000000000000000000, -1.000000000000000000 ) ) ;
#2942=ORIENTED_EDGE ( 'NONE', *, *, #9479, .F. ) ;
#2947=DIRECTION ( 'NONE',  ( -1.000000000000000000, 0.000000000000000000, 0.000000000000000000 ) ) ;
#2949=DIRECTION ( 'NONE',  ( -1.000000000000000000, 0.000000000000000000, 0.000000000000000000 ) ) ;
#2953=VERTEX_POINT ( 'NONE', #4915 ) ;
#2957=DIRECTION ( 'NONE',  ( 0.000000000000000000, 0.000000000000000000, 1.000000000000000000 ) ) ;
#2958=VERTEX_POINT ( 'NONE', #618 ) ;
#2961=ORIENTED_EDGE ( 'NONE', *, *, #8615, .F. ) ;
#2962=B_SPLINE_CURVE_WITH_KNOTS ( 'NONE', 3,
 ( #8531, #908, #9241, #4134, #2525, #4309, #7755, #7698, #3478, #7522, #6859, #2652, #6027, #10912, #4368, #6688, #9411, #8409 ),
 .UNSPECIFIED., .F., .F.,
 ( 4, 2, 2, 2, 2, 2, 2, 2, 4 ),
 ( 0.000000000000000000, 0.0005875687307069784411, 0.001175137461413956882, 0.001762706192120935648, 0.002350274922827915065, 0.002937843653534894482, 0.003525412384241873899, 0.004112981114948852449, 0.004700549845655830998 ),
 .UNSPECIFIED. ) ;
#2970=LINE ( 'NONE', #1236, #672 ) ;
#2971=CYLINDRICAL_SURFACE ( 'NONE', #5952, 2.149999999999988809 ) ;
#2973=VERTEX_POINT ( 'NONE', #10900 ) ;
#2974=ORIENTED_EDGE ( 'NONE', *, *, #3498, .T. ) ;
#2980=VECTOR ( 'NONE', #517, 1000.000000000000000 ) ;
#2989=AXIS2_PLACEMENT_3D ( 'NONE', #9579, #241, #6242 ) ;
#2997=CARTESIAN_POINT ( 'NONE',  ( -25.71106610644865498, 16.50000000000026290, -9.500000000000000000 ) ) ;
#3002=ORIENTED_EDGE ( 'NONE', *, *, #761, .T. ) ;
#3008=CARTESIAN_POINT ( 'NONE',  ( 34.85586774767502050, 3.177316488306994646, 3.109148447068123655 ) ) ;
#3010=LINE ( 'NONE', #1903, #3330 ) ;
#3022=DIRECTION ( 'NONE',  ( -1.000000000000000000, 0.000000000000000000, 0.000000000000000000 ) ) ;
#3023=EDGE_LOOP ( 'NONE', ( #9776, #1790, #2325, #7797 ) ) ;
#3033=ORIENTED_EDGE ( 'NONE', *, *, #242, .F. ) ;
#3043=DIRECTION ( 'NONE',  ( 0.000000000000000000, 0.000000000000000000, 1.000000000000000000 ) ) ;
#3045=CIRCLE ( 'NONE', #9239, 3.000000000000000000 ) ;
#3049=ORIENTED_EDGE ( 'NONE', *, *, #2342, .F. ) ;
#3050=ADVANCED_FACE ( 'NONE', ( #984 ), #2884, .F. ) ;
#3052=VECTOR ( 'NONE', #2515, 999.9999999999998863 ) ;
#3071=ORIENTED_EDGE ( 'NONE', *, *, #6203, .F. ) ;
#3095=VERTEX_POINT ( 'NONE', #7827 ) ;
#3099=CARTESIAN_POINT ( 'NONE',  ( 0.000000000000000000, 0.000000000000000000, -9.500000000000000000 ) ) ;
#3106=CARTESIAN_POINT ( 'NONE',  ( 34.76670834929980458, 4.038474554490623980, 2.651503408690715435 ) ) ;
#3112=VECTOR ( 'NONE', #3435, 1000.000000000000000 ) ;
#3132=DIRECTION ( 'NONE',  ( -0.000000000000000000, -0.000000000000000000, 1.000000000000000000 ) ) ;
#3137=DIRECTION ( 'NONE',  ( 1.000000000000000000, 6.098637220230964906E-17, 0.000000000000000000 ) ) ;
#3142=CYLINDRICAL_SURFACE ( 'NONE', #446, 3.000000000000000000 ) ;
#3145=COLOUR_RGB ( '', 0.08235294, 0.09019608, 0.10196078) ;
#3160=VERTEX_POINT ( 'NONE', #5497 ) ;
#3205=ADVANCED_FACE ( 'NONE', ( #8150 ), #3142, .F. ) ;
#3207=ORIENTED_EDGE ( 'NONE', *, *, #793, .T. ) ;
#3214=VECTOR ( 'NONE', #188, 1000.000000000000000 ) ;
#3218=DIRECTION ( 'NONE',  ( 4.312387734421999162E-17, -0.7071067811865487940, 0.7071067811865463515 ) ) ;
#3229=EDGE_LOOP ( 'NONE', ( #6223, #10215, #2667, #9993 ) ) ;
#3234=CARTESIAN_POINT ( 'NONE',  ( -30.75045812061784289, 13.49999999999941913, -2.500000000000000000 ) ) ;
#3237=CARTESIAN_POINT ( 'NONE',  ( 34.99999999999999289, -3.999999999999993339, 7.850000000000016520 ) ) ;
#3244=CARTESIAN_POINT ( 'NONE',  ( -25.98076211353324894, 14.99999999999984190, -2.500000000000000000 ) ) ;
#3247=DIRECTION ( 'NONE',  ( -1.000000000000000000, 0.000000000000000000, 0.000000000000000000 ) ) ;
#3251=DIRECTION ( 'NONE',  ( 0.000000000000000000, 0.000000000000000000, -1.000000000000000000 ) ) ;
#3252=CARTESIAN_POINT ( 'NONE',  ( -25.98076211353324894, 14.99999999999984190, 2.500000000000000000 ) ) ;
#3261=ORIENTED_EDGE ( 'NONE', *, *, #7499, .F. ) ;
#3264=PLANE ( 'NONE',  #1488 ) ;
#3273=CLOSED_SHELL ( 'NONE', ( #8289, #9821, #360, #167, #2502, #545, #6210, #6896, #10094, #7838, #5815, #589, #1948, #4252, #33, #5604, #5660, #4014, #8170, #5864, #10955, #9080, #3832, #49, #3205, #6975, #10069, #9446, #7435, #2612, #1520, #1865, #8528, #3425, #2070, #6690, #4370, #3050, #7009, #7711, #8496, #6925, #4383 ) ) ;
#3284=AXIS2_PLACEMENT_3D ( 'NONE', #6497, #1452, #3949 ) ;
#3288=ORIENTED_EDGE ( 'NONE', *, *, #573, .F. ) ;
#3291=EDGE_CURVE ( 'NONE', #7662, #6545, #9864, .T. ) ;
#3301=ORIENTED_EDGE ( 'NONE', *, *, #8526, .T. ) ;
#3308=CYLINDRICAL_SURFACE ( 'NONE', #1615, 1.500000000000001332 ) ;
#3310=DIRECTION ( 'NONE',  ( -0.000000000000000000, 1.000000000000000000, -0.000000000000000000 ) ) ;
#3314=CARTESIAN_POINT ( 'NONE',  ( 29.49999999999999289, -9.999999999999998224, 15.50000000000000533 ) ) ;
#3330=VECTOR ( 'NONE', #5289, 1000.000000000000000 ) ;
#3345=AXIS2_PLACEMENT_3D ( 'NONE', #5480, #4436, #1613 ) ;
#3358=EDGE_CURVE ( 'NONE', #3095, #1804, #2402, .T. ) ;
#3359=ORIENTED_EDGE ( 'NONE', *, *, #1117, .T. ) ;
#3360=ORIENTED_EDGE ( 'NONE', *, *, #3422, .T. ) ;
#3362=DIRECTION ( 'NONE',  ( -0.000000000000000000, 0.000000000000000000, -1.000000000000000000 ) ) ;
#3368=LINE ( 'NONE', #9471, #4589 ) ;
#3373=CARTESIAN_POINT ( 'NONE',  ( 24.30992024302470256, 5.833333333333333925, 2.500000000000000000 ) ) ;
#3380=ORIENTED_EDGE ( 'NONE', *, *, #9822, .T. ) ;
#3385=VERTEX_POINT ( 'NONE', #2482 ) ;
#3386=CARTESIAN_POINT ( 'NONE',  ( 29.49999999999999289, 2.000000000000001776, 5.500000000000000000 ) ) ;
#3388=ORIENTED_EDGE ( 'NONE', *, *, #4917, .F. ) ;
#3395=AXIS2_PLACEMENT_3D ( 'NONE', #6191, #3538, #1977 ) ;
#3403=VECTOR ( 'NONE', #10846, 1000.000000000000000 ) ;
#3417=PRODUCT ( 'caliper arm right', 'caliper arm right', '', ( #7210 ) ) ;
#3422=EDGE_CURVE ( 'NONE', #4007, #9236, #6751, .T. ) ;
#3425=ADVANCED_FACE ( 'NONE', ( #9367 ), #1078, .T. ) ;
#3429=VERTEX_POINT ( 'NONE', #7037 ) ;
#3434=EDGE_CURVE ( 'NONE', #3095, #8941, #3542, .T. ) ;
#3435=DIRECTION ( 'NONE',  ( 0.000000000000000000, 0.000000000000000000, 1.000000000000000000 ) ) ;
#3456=CARTESIAN_POINT ( 'NONE',  ( -25.98076211353324894, 14.99999999999984190, 2.500000000000000000 ) ) ;
#3457=EDGE_LOOP ( 'NONE', ( #9378, #4513, #10645, #2408 ) ) ;
#3462=ORIENTED_EDGE ( 'NONE', *, *, #8656, .T. ) ;
#3478=CARTESIAN_POINT ( 'NONE',  ( 34.89259351528886555, 2.743407123163640104, -3.513512538347002057 ) ) ;
#3492=DIRECTION ( 'NONE',  ( 0.000000000000000000, 0.000000000000000000, 1.000000000000000000 ) ) ;
#3498=EDGE_CURVE ( 'NONE', #9249, #7102, #191, .T. ) ;
#3510=EDGE_CURVE ( 'NONE', #9249, #5721, #2761, .T. ) ;
#3511=DIRECTION ( 'NONE',  ( -1.000000000000000000, 0.000000000000000000, 0.000000000000000000 ) ) ;
#3521=VECTOR ( 'NONE', #5451, 1000.000000000000000 ) ;
#3529=VERTEX_POINT ( 'NONE', #1930 ) ;
#3538=DIRECTION ( 'NONE',  ( 0.000000000000000000, -1.000000000000000000, -0.000000000000000000 ) ) ;
#3542=LINE ( 'NONE', #9530, #1158 ) ;
#3544=LINE ( 'NONE', #3645, #6703 ) ;
#3588=LINE ( 'NONE', #8025, #6306 ) ;
#3601=CARTESIAN_POINT ( 'NONE',  ( -30.75045812061784289, 16.50000000000026290, -5.000000000000000000 ) ) ;
#3617=VERTEX_POINT ( 'NONE', #10687 ) ;
#3622=VECTOR ( 'NONE', #7720, 1000.000000000000000 ) ;
#3627=LINE ( 'NONE', #10350, #6473 ) ;
#3629=ORIENTED_EDGE ( 'NONE', *, *, #1622, .F. ) ;
#3630=EDGE_CURVE ( 'NONE', #3617, #1228, #10736, .T. ) ;
#3631=ORIENTED_EDGE ( 'NONE', *, *, #9460, .T. ) ;
#3634=DIRECTION ( 'NONE',  ( -0.000000000000000000, -1.000000000000000000, -0.000000000000000000 ) ) ;
#3640=DIRECTION ( 'NONE',  ( 1.000000000000000000, 0.000000000000000000, 0.000000000000000000 ) ) ;
#3643=CARTESIAN_POINT ( 'NONE',  ( 5.076455387921338769, 24.47916666666667140, 0.000000000000000000 ) ) ;
#3645=CARTESIAN_POINT ( 'NONE',  ( -30.75045812061784289, 16.50000000000026290, -9.500000000000000000 ) ) ;
#3646=AXIS2_PLACEMENT_3D ( 'NONE', #6324, #5386, #8771 ) ;
#3652=DIRECTION ( 'NONE',  ( 0.000000000000000000, 0.000000000000000000, -1.000000000000000000 ) ) ;
#3656=CARTESIAN_POINT ( 'NONE',  ( 34.99999999999999289, -3.999999999999993339, -4.999999999999995559 ) ) ;
#3674=ORIENTED_EDGE ( 'NONE', *, *, #4582, .F. ) ;
#3688=CYLINDRICAL_SURFACE ( 'NONE', #5620, 5.000000000000000888 ) ;
#3690=AXIS2_PLACEMENT_3D ( 'NONE', #10631, #7858, #3022 ) ;
#3700=CARTESIAN_POINT ( 'NONE',  ( 34.99999999999999289, 2.000000000000002220, -12.49999999999999822 ) ) ;
#3710=CARTESIAN_POINT ( 'NONE',  ( 6.015568632492056977, 34.47916666666665009, 2.500000000000000000 ) ) ;
#3723=VERTEX_POINT ( 'NONE', #1361 ) ;
#3726=DIRECTION ( 'NONE',  ( -1.000000000000000000, 0.000000000000000000, 0.000000000000000000 ) ) ;
#3737=CARTESIAN_POINT ( 'NONE',  ( -1.219727444046192735E-16, 2.000000000000000000, -10.50000000000000355 ) ) ;
#3738=DIRECTION ( 'NONE',  ( -1.000000000000000000, -6.098637220230963674E-17, -1.156482317317871725E-16 ) ) ;
#3745=FACE_OUTER_BOUND ( 'NONE', #10501, .T. ) ;
#3748=CARTESIAN_POINT ( 'NONE',  ( 34.99999999999999289, -9.999999999999998224, -10.50000000000000355 ) ) ;
#3756=CIRCLE ( 'NONE', #6617, 2.149999999999987921 ) ;
#3771=EDGE_CURVE ( 'NONE', #10326, #8941, #1173, .T. ) ;
#3773=ORIENTED_EDGE ( 'NONE', *, *, #2201, .F. ) ;
#3786=ORIENTED_EDGE ( 'NONE', *, *, #1898, .F. ) ;
#3804=AXIS2_PLACEMENT_3D ( 'NONE', #6259, #4557, #2048 ) ;
#3832=ADVANCED_FACE ( 'NONE', ( #2468 ), #1684, .F. ) ;
#3848=FACE_OUTER_BOUND ( 'NONE', #4967, .T. ) ;
#3850=ORIENTED_EDGE ( 'NONE', *, *, #7228, .T. ) ;
#3855=VECTOR ( 'NONE', #3132, 1000.000000000000000 ) ;
#3870=DIRECTION ( 'NONE',  ( -0.000000000000000000, -0.000000000000000000, -1.000000000000000000 ) ) ;
#3880=( GEOMETRIC_REPRESENTATION_CONTEXT ( 3 ) GLOBAL_UNCERTAINTY_ASSIGNED_CONTEXT ( ( #515 ) ) GLOBAL_UNIT_ASSIGNED_CONTEXT ( ( #7040, #8589, #4098 ) ) REPRESENTATION_CONTEXT ( 'NONE', 'WORKASPACE' ) );
#3881=DIRECTION ( 'NONE',  ( -0.000000000000000000, -0.000000000000000000, -1.000000000000000000 ) ) ;
#3885=VERTEX_POINT ( 'NONE', #7575 ) ;
#3889=ORIENTED_EDGE ( 'NONE', *, *, #1459, .T. ) ;
#3906=CARTESIAN_POINT ( 'NONE',  ( 34.99999999999999289, -3.999999999999993339, -7.149999999999987921 ) ) ;
#3914=CARTESIAN_POINT ( 'NONE',  ( -1.219727444046192735E-16, 2.000000000000000000, 0.000000000000000000 ) ) ;
#3919=CYLINDRICAL_SURFACE ( 'NONE', #10740, 2.649999999999991029 ) ;
#3924=AXIS2_PLACEMENT_3D ( 'NONE', #2465, #5847, #9230 ) ;
#3925=ORIENTED_EDGE ( 'NONE', *, *, #603, .T. ) ;
#3930=DIRECTION ( 'NONE',  ( -1.000000000000000000, 0.000000000000000000, 0.000000000000000000 ) ) ;
#3949=DIRECTION ( 'NONE',  ( -1.000000000000000000, 0.000000000000000000, 0.000000000000000000 ) ) ;
#3970=AXIS2_PLACEMENT_3D ( 'NONE', #9320, #929, #2493 ) ;
#3977=AXIS2_PLACEMENT_3D ( 'NONE', #4394, #6716, #7781 ) ;
#3978=DIRECTION ( 'NONE',  ( 0.000000000000000000, 0.000000000000000000, 1.000000000000000000 ) ) ;
#3980=CIRCLE ( 'NONE', #10384, 7.500000000000000000 ) ;
#3985=CARTESIAN_POINT ( 'NONE',  ( 29.49999999999999645, -9.999999999999998224, -12.49999999999999822 ) ) ;
#3987=EDGE_CURVE ( 'NONE', #9988, #3885, #9512, .T. ) ;
#3996=VECTOR ( 'NONE', #10258, 1000.000000000000000 ) ;
#4007=VERTEX_POINT ( 'NONE', #8821 ) ;
#4014=ADVANCED_FACE ( 'NONE', ( #9646 ), #6467, .T. ) ;
#4019=ORIENTED_EDGE ( 'NONE', *, *, #9675, .T. ) ;
#4037=FACE_OUTER_BOUND ( 'NONE', #2439, .T. ) ;
#4040=VECTOR ( 'NONE', #5781, 1000.000000000000000 ) ;
#4049=ORIENTED_EDGE ( 'NONE', *, *, #624, .T. ) ;
#4051=CARTESIAN_POINT ( 'NONE',  ( -26.25045812061784289, 13.49999999999941913, -9.500000000000000000 ) ) ;
#4052=ORIENTED_EDGE ( 'NONE', *, *, #6268, .F. ) ;
#4078=ORIENTED_EDGE ( 'NONE', *, *, #4312, .F. ) ;
#4098=( NAMED_UNIT ( * ) SI_UNIT ( $, .STERADIAN. ) SOLID_ANGLE_UNIT ( ) );
#4101=ORIENTED_EDGE ( 'NONE', *, *, #421, .F. ) ;
#4112=CARTESIAN_POINT ( 'NONE',  ( 34.99999999999999289, -9.999999999999998224, -10.50000000000000355 ) ) ;
#4122=CARTESIAN_POINT ( 'NONE',  ( 34.99999999999999289, -3.999999999999993339, 12.14999999999999503 ) ) ;
#4127=CARTESIAN_POINT ( 'NONE',  ( 0.000000000000000000, 0.000000000000000000, 2.500000000000000000 ) ) ;
#4134=CARTESIAN_POINT ( 'NONE',  ( 34.93719828579781250, 2.096102678619138793, -4.721690477507366701 ) ) ;
#4140=ORIENTED_EDGE ( 'NONE', *, *, #5357, .T. ) ;
#4168=AXIS2_PLACEMENT_3D ( 'NONE', #1616, #1731, #942 ) ;
#4170=DIRECTION ( 'NONE',  ( -0.000000000000000000, 1.000000000000000000, -0.000000000000000000 ) ) ;
#4173=ORIENTED_EDGE ( 'NONE', *, *, #3630, .T. ) ;
#4174=VECTOR ( 'NONE', #2913, 1000.000000000000000 ) ;
#4180=EDGE_CURVE ( 'NONE', #609, #1386, #5437, .T. ) ;
#4188=CARTESIAN_POINT ( 'NONE',  ( -25.98076211353324894, 16.50000000000026290, -2.850000000000009859 ) ) ;
#4190=EDGE_CURVE ( 'NONE', #6778, #10326, #4737, .T. ) ;
#4193=CARTESIAN_POINT ( 'NONE',  ( -25.98076211353324894, 14.99999999999984190, -2.500000000000000000 ) ) ;
#4202=DIRECTION ( 'NONE',  ( -1.000000000000000000, 0.000000000000000000, 0.000000000000000000 ) ) ;
#4205=PLANE ( 'NONE',  #8059 ) ;
#4212=AXIS2_PLACEMENT_3D ( 'NONE', #9861, #622, #5853 ) ;
#4218=CARTESIAN_POINT ( 'NONE',  ( -30.98076211353324894, 14.99999999999984190, 2.500000000000000000 ) ) ;
#4220=FACE_OUTER_BOUND ( 'NONE', #8046, .T. ) ;
#4235=ORIENTED_EDGE ( 'NONE', *, *, #5215, .T. ) ;
#4240=ORIENTED_EDGE ( 'NONE', *, *, #253, .T. ) ;
#4252=ADVANCED_FACE ( 'NONE', ( #1636 ), #785, .T. ) ;
#4265=LINE ( 'NONE', #7651, #1856 ) ;
#4275=CARTESIAN_POINT ( 'NONE',  ( -25.98076211353324894, 16.50000000000026290, -2.850000000000008082 ) ) ;
#4288=CARTESIAN_POINT ( 'NONE',  ( -25.98076211353324894, 16.50000000000026290, -5.000000000000000000 ) ) ;
#4289=ORIENTED_EDGE ( 'NONE', *, *, #9663, .T. ) ;
#4290=AXIS2_PLACEMENT_3D ( 'NONE', #3456, #9443, #3511 ) ;
#4296=DIRECTION ( 'NONE',  ( 0.000000000000000000, 0.000000000000000000, 1.000000000000000000 ) ) ;
#4300=CARTESIAN_POINT ( 'NONE',  ( -26.25045812061784289, 0.000000000000000000, -9.500000000000000000 ) ) ;
#4305=VERTEX_POINT ( 'NONE', #7970 ) ;
#4309=CARTESIAN_POINT ( 'NONE',  ( 34.92408131826246631, 2.305272916965852570, -4.166859826334558647 ) ) ;
#4312=EDGE_CURVE ( 'NONE', #1351, #6840, #1857, .T. ) ;
#4320=CARTESIAN_POINT ( 'NONE',  ( -25.71106610644865498, 13.49999999999941913, -9.500000000000000000 ) ) ;
#4336=DIRECTION ( 'NONE',  ( -0.000000000000000000, 1.000000000000000000, -0.000000000000000000 ) ) ;
#4346=EDGE_LOOP ( 'NONE', ( #8114, #5498, #4049, #8317 ) ) ;
#4360=CIRCLE ( 'NONE', #10567, 2.649999999999992362 ) ;
#4363=ORIENTED_EDGE ( 'NONE', *, *, #2625, .F. ) ;
#4368=CARTESIAN_POINT ( 'NONE',  ( 34.74482695545609801, 4.223122737142881000, -2.595677240809972641 ) ) ;
#4370=ADVANCED_FACE ( 'NONE', ( #4429 ), #4526, .T. ) ;
#4374=DIRECTION ( 'NONE',  ( -1.000000000000000000, -6.098637220230964906E-17, 0.000000000000000000 ) ) ;
#4382=APPLICATION_CONTEXT ( 'automotive_design' ) ;
#4383=ADVANCED_FACE ( 'NONE', ( #7082 ), #3688, .T. ) ;
#4392=FACE_OUTER_BOUND ( 'NONE', #730, .T. ) ;
#4394=CARTESIAN_POINT ( 'NONE',  ( 0.000000000000000000, 0.000000000000000000, 2.500000000000000000 ) ) ;
#4398=CARTESIAN_POINT ( 'NONE',  ( 34.99999999999999289, -3.999999999999993339, -2.850000000000003642 ) ) ;
#4423=CARTESIAN_POINT ( 'NONE',  ( 29.49999999999999289, -3.999999999999993339, 7.850000000000016520 ) ) ;
#4429=FACE_OUTER_BOUND ( 'NONE', #203, .T. ) ;
#4436=DIRECTION ( 'NONE',  ( 0.000000000000000000, 1.000000000000000000, 0.000000000000000000 ) ) ;
#4437=DIRECTION ( 'NONE',  ( -6.308085367188384325E-16, -3.847072420872938447E-32, 1.000000000000000000 ) ) ;
#4446=CARTESIAN_POINT ( 'NONE',  ( 34.99999999999999289, 2.000000000000002220, -10.50000000000000355 ) ) ;
#4463=VERTEX_POINT ( 'NONE', #8552 ) ;
#4478=ORIENTED_EDGE ( 'NONE', *, *, #5357, .F. ) ;
#4494=CARTESIAN_POINT ( 'NONE',  ( 29.17190429162963738, 2.000000000000001776, -12.50099999999999767 ) ) ;
#4513=ORIENTED_EDGE ( 'NONE', *, *, #2602, .F. ) ;
#4515=VERTEX_POINT ( 'NONE', #519 ) ;
#4526=PLANE ( 'NONE',  #2785 ) ;
#4531=CIRCLE ( 'NONE', #8611, 24.99999999999999645 ) ;
#4539=DIRECTION ( 'NONE',  ( -0.000000000000000000, -0.000000000000000000, -1.000000000000000000 ) ) ;
#4540=ORIENTED_EDGE ( 'NONE', *, *, #2856, .T. ) ;
#4541=DIRECTION ( 'NONE',  ( 0.000000000000000000, 1.000000000000000000, 0.000000000000000000 ) ) ;
#4547=CARTESIAN_POINT ( 'NONE',  ( -25.98076211353324894, 13.49999999999941913, -2.850000000000009859 ) ) ;
#4554=VECTOR ( 'NONE', #4539, 1000.000000000000000 ) ;
#4556=ORIENTED_EDGE ( 'NONE', *, *, #1898, .T. ) ;
#4557=DIRECTION ( 'NONE',  ( 0.000000000000000000, 1.000000000000000000, 0.000000000000000000 ) ) ;
#4582=EDGE_CURVE ( 'NONE', #10904, #7860, #9919, .T. ) ;
#4583=VERTEX_POINT ( 'NONE', #5696 ) ;
#4585=EDGE_CURVE ( 'NONE', #143, #9227, #9495, .T. ) ;
#4588=DIRECTION ( 'NONE',  ( -1.000000000000000000, 0.000000000000000000, 0.000000000000000000 ) ) ;
#4589=VECTOR ( 'NONE', #4374, 1000.000000000000000 ) ;
#4634=LINE ( 'NONE', #2076, #1010 ) ;
#4642=LINE ( 'NONE', #7290, #6230 ) ;
#4646=EDGE_LOOP ( 'NONE', ( #6823, #7487 ) ) ;
#4647=CARTESIAN_POINT ( 'NONE',  ( 29.49999999999999645, 2.000000000000001776, -12.49999999999999822 ) ) ;
#4655=DIRECTION ( 'NONE',  ( -0.000000000000000000, -1.000000000000000000, -0.000000000000000000 ) ) ;
#4663=DIRECTION ( 'NONE',  ( 0.000000000000000000, 0.000000000000000000, 1.000000000000000000 ) ) ;
#4669=VECTOR ( 'NONE', #8200, 1000.000000000000000 ) ;
#4696=FACE_OUTER_BOUND ( 'NONE', #5927, .T. ) ;
#4700=CARTESIAN_POINT ( 'NONE',  ( 34.99999999999999289, 1.000000000000004663, -11.50000000000000533 ) ) ;
#4734=ORIENTED_EDGE ( 'NONE', *, *, #10918, .F. ) ;
#4737=CIRCLE ( 'NONE', #5779, 4.999999999999997335 ) ;
#4771=COLOUR_RGB ( '', 0.08235294, 0.09019608, 0.10196078) ;
#4777=VERTEX_POINT ( 'NONE', #1580 ) ;
#4810=CARTESIAN_POINT ( 'NONE',  ( 21.55579831881754416, 20.86490736922957367, 2.500000000000000444 ) ) ;
#4820=PLANE ( 'NONE',  #9622 ) ;
#4827=DIRECTION ( 'NONE',  ( 1.000000000000000000, 0.000000000000000000, -0.000000000000000000 ) ) ;
#4834=EDGE_LOOP ( 'NONE', ( #5881, #4919, #5560, #1551, #3071, #8100 ) ) ;
#4835=CARTESIAN_POINT ( 'NONE',  ( 29.49999999999999645, -3.999999999999993339, -7.149999999999983480 ) ) ;
#4836=ORIENTED_EDGE ( 'NONE', *, *, #5735, .T. ) ;
#4874=LINE ( 'NONE', #7368, #4669 ) ;
#4889=ORIENTED_EDGE ( 'NONE', *, *, #3510, .T. ) ;
#4894=VECTOR ( 'NONE', #1528, 1000.000000000000000 ) ;
#4899=FACE_OUTER_BOUND ( 'NONE', #5052, .T. ) ;
#4915=CARTESIAN_POINT ( 'NONE',  ( 29.17190429162964094, 2.000000000000001776, 2.500000000000000000 ) ) ;
#4917=EDGE_CURVE ( 'NONE', #10021, #6926, #2812, .T. ) ;
#4919=ORIENTED_EDGE ( 'NONE', *, *, #1594, .T. ) ;
#4920=CARTESIAN_POINT ( 'NONE',  ( -25.98076211353324894, 14.99999999999984190, 2.500000000000000000 ) ) ;
#4921=EDGE_CURVE ( 'NONE', #5409, #9236, #9520, .T. ) ;
#4934=DIRECTION ( 'NONE',  ( 0.000000000000000000, 0.000000000000000000, 1.000000000000000000 ) ) ;
#4935=EDGE_LOOP ( 'NONE', ( #10605, #3629, #5753, #3786 ) ) ;
#4942=VECTOR ( 'NONE', #1791, 1000.000000000000114 ) ;
#4950=ORIENTED_EDGE ( 'NONE', *, *, #4180, .F. ) ;
#4967=EDGE_LOOP ( 'NONE', ( #8207, #2372, #2809, #9753, #9597, #495, #5345, #4478, #1381, #9121, #10111, #1067, #1112, #7707, #9001 ) ) ;
#4970=LINE ( 'NONE', #4122, #9736 ) ;
#4973=DIRECTION ( 'NONE',  ( -1.000000000000000000, 0.000000000000000000, 0.000000000000000000 ) ) ;
#4977=ORIENTED_EDGE ( 'NONE', *, *, #3630, .F. ) ;
#4987=DIRECTION ( 'NONE',  ( -0.000000000000000000, -0.000000000000000000, 1.000000000000000000 ) ) ;
#4996=EDGE_LOOP ( 'NONE', ( #10275, #4289, #9183, #1653 ) ) ;
#5013=CARTESIAN_POINT ( 'NONE',  ( -25.98076211353324894, 16.50000000000026290, -7.149999999999992362 ) ) ;
#5019=CIRCLE ( 'NONE', #6783, 1.500000000000001332 ) ;
#5024=DIRECTION ( 'NONE',  ( 1.000000000000000000, -0.000000000000000000, -0.000000000000000000 ) ) ;
#5029=FACE_OUTER_BOUND ( 'NONE', #9394, .T. ) ;
#5034=CARTESIAN_POINT ( 'NONE',  ( 34.99999999999999289, -7.999999999999996447, 17.50000000000000355 ) ) ;
#5038=DIRECTION ( 'NONE',  ( -1.000000000000000000, 0.000000000000000000, 0.000000000000000000 ) ) ;
#5046=AXIS2_PLACEMENT_3D ( 'NONE', #8491, #752, #10162 ) ;
#5048=CARTESIAN_POINT ( 'NONE',  ( 34.99999999999999289, -3.999999999999993339, -4.999999999999995559 ) ) ;
#5052=EDGE_LOOP ( 'NONE', ( #7337, #3033, #4977, #1066 ) ) ;
#5059=VERTEX_POINT ( 'NONE', #865 ) ;
#5097=PLANE ( 'NONE',  #7906 ) ;
#5101=CARTESIAN_POINT ( 'NONE',  ( -30.75045812061784289, 13.49999999999941913, -9.500000000000000000 ) ) ;
#5109=( GEOMETRIC_REPRESENTATION_CONTEXT ( 3 ) GLOBAL_UNCERTAINTY_ASSIGNED_CONTEXT ( ( #18 ) ) GLOBAL_UNIT_ASSIGNED_CONTEXT ( ( #5479, #8867, #10586 ) ) REPRESENTATION_CONTEXT ( 'NONE', 'WORKASPACE' ) );
#5111=ORIENTED_EDGE ( 'NONE', *, *, #7191, .T. ) ;
#5113=DIRECTION ( 'NONE',  ( 1.000000000000000000, 6.098637220230964906E-17, 0.000000000000000000 ) ) ;
#5115=CYLINDRICAL_SURFACE ( 'NONE', #7718, 2.649999999999991029 ) ;
#5121=DIRECTION ( 'NONE',  ( -1.000000000000000000, 0.000000000000000000, 0.000000000000000000 ) ) ;
#5141=DIRECTION ( 'NONE',  ( -1.000000000000000000, 0.000000000000000000, 0.000000000000000000 ) ) ;
#5143=DIRECTION ( 'NONE',  ( 1.000000000000000000, -0.000000000000000000, -0.000000000000000000 ) ) ;
#5154=CARTESIAN_POINT ( 'NONE',  ( -6.015568632492056977, 34.47916666666665009, 2.500000000000000000 ) ) ;
#5156=DIRECTION ( 'NONE',  ( -0.000000000000000000, -0.000000000000000000, 1.000000000000000000 ) ) ;
#5158=DIRECTION ( 'NONE',  ( 0.000000000000000000, 0.000000000000000000, -1.000000000000000000 ) ) ;
#5165=VERTEX_POINT ( 'NONE', #7932 ) ;
#5214=EDGE_CURVE ( 'NONE', #3160, #1491, #8485, .T. ) ;
#5215=EDGE_CURVE ( 'NONE', #6853, #2434, #9457, .T. ) ;
#5232=FACE_OUTER_BOUND ( 'NONE', #1971, .T. ) ;
#5233=ORIENTED_EDGE ( 'NONE', *, *, #9761, .T. ) ;
#5235=ORIENTED_EDGE ( 'NONE', *, *, #6626, .F. ) ;
#5244=AXIS2_PLACEMENT_3D ( 'NONE', #7058, #268, #2949 ) ;
#5261=CARTESIAN_POINT ( 'NONE',  ( 29.49999999999999289, 2.000000000000001776, -12.50099999999999767 ) ) ;
#5262=ORIENTED_EDGE ( 'NONE', *, *, #2738, .T. ) ;
#5269=LINE ( 'NONE', #803, #3112 ) ;
#5273=CARTESIAN_POINT ( 'NONE',  ( -30.31088913245546124, 17.49999999999980815, -2.500000000000000000 ) ) ;
#5289=DIRECTION ( 'NONE',  ( -0.000000000000000000, -0.000000000000000000, -1.000000000000000000 ) ) ;
#5295=ORIENTED_EDGE ( 'NONE', *, *, #555, .F. ) ;
#5303=DIRECTION ( 'NONE',  ( 1.000000000000000000, -0.000000000000000000, -0.000000000000000000 ) ) ;
#5306=ORIENTED_EDGE ( 'NONE', *, *, #7454, .F. ) ;
#5325=DIRECTION ( 'NONE',  ( -1.000000000000000000, -6.098637220230964906E-17, -6.308085367188384325E-16 ) ) ;
#5342=LINE ( 'NONE', #331, #6887 ) ;
#5345=ORIENTED_EDGE ( 'NONE', *, *, #838, .F. ) ;
#5354=LINE ( 'NONE', #231, #4174 ) ;
#5356=VERTEX_POINT ( 'NONE', #7855 ) ;
#5357=EDGE_CURVE ( 'NONE', #3529, #2609, #2970, .T. ) ;
#5360=CARTESIAN_POINT ( 'NONE',  ( 0.000000000000000000, 30.00000000000000000, -2.499999999999998668 ) ) ;
#5364=DIRECTION ( 'NONE',  ( -1.000000000000000000, 0.000000000000000000, 0.000000000000000000 ) ) ;
#5386=DIRECTION ( 'NONE',  ( 1.000000000000000000, 6.098637220230963674E-17, 1.156482317317871725E-16 ) ) ;
#5389=ORIENTED_EDGE ( 'NONE', *, *, #5876, .F. ) ;
#5397=ORIENTED_EDGE ( 'NONE', *, *, #2625, .T. ) ;
#5409=VERTEX_POINT ( 'NONE', #1331 ) ;
#5415=CIRCLE ( 'NONE', #3646, 3.000000000000000888 ) ;
#5424=EDGE_LOOP ( 'NONE', ( #5111, #2472 ) ) ;
#5433=AXIS2_PLACEMENT_3D ( 'NONE', #8697, #6132, #8803 ) ;
#5437=CIRCLE ( 'NONE', #628, 4.500000000000000000 ) ;
#5451=DIRECTION ( 'NONE',  ( -6.098637220230963674E-17, 1.000000000000000000, 0.000000000000000000 ) ) ;
#5467=EDGE_CURVE ( 'NONE', #8941, #5409, #10447, .T. ) ;
#5477=DIRECTION ( 'NONE',  ( -0.000000000000000000, 1.000000000000000000, -0.000000000000000000 ) ) ;
#5479=( LENGTH_UNIT ( ) NAMED_UNIT ( * ) SI_UNIT ( .MILLI., .METRE. ) );
#5480=CARTESIAN_POINT ( 'NONE',  ( -21.21106610644865498, 13.49999999999941913, -9.500000000000000000 ) ) ;
#5486=EDGE_CURVE ( 'NONE', #6952, #10021, #6694, .T. ) ;
#5493=EDGE_CURVE ( 'NONE', #7488, #8716, #1280, .T. ) ;
#5497=CARTESIAN_POINT ( 'NONE',  ( 34.64101615137754209, 5.000000000000001776, -2.500000000000000000 ) ) ;
#5498=ORIENTED_EDGE ( 'NONE', *, *, #8266, .T. ) ;
#5504=LINE ( 'NONE', #1277, #267 ) ;
#5510=ORIENTED_EDGE ( 'NONE', *, *, #10557, .F. ) ;
#5513=EDGE_LOOP ( 'NONE', ( #2284, #6652, #1226, #3360 ) ) ;
#5522=ORIENTED_EDGE ( 'NONE', *, *, #7228, .F. ) ;
#5550=EDGE_CURVE ( 'NONE', #1351, #5059, #3544, .T. ) ;
#5557=ORIENTED_EDGE ( 'NONE', *, *, #6626, .T. ) ;
#5559=MANIFOLD_SOLID_BREP ( 'Fillet4', #3273 ) ;
#5560=ORIENTED_EDGE ( 'NONE', *, *, #5550, .T. ) ;
#5592=AXIS2_PLACEMENT_3D ( 'NONE', #8102, #480, #3930 ) ;
#5600=VECTOR ( 'NONE', #10676, 1000.000000000000000 ) ;
#5604=ADVANCED_FACE ( 'NONE', ( #7195, #9754, #1255 ), #10931, .T. ) ;
#5620=AXIS2_PLACEMENT_3D ( 'NONE', #7753, #10356, #6025 ) ;
#5635=AXIS2_PLACEMENT_3D ( 'NONE', #4127, #9071, #8402 ) ;
#5639=CARTESIAN_POINT ( 'NONE',  ( 0.000000000000000000, 0.000000000000000000, 2.500000000000000000 ) ) ;
#5660=ADVANCED_FACE ( 'NONE', ( #9805, #8813, #10482 ), #7930, .T. ) ;
#5667=CARTESIAN_POINT ( 'NONE',  ( 34.69563600136375214, 4.609751841799208272, 2.519143709543159471 ) ) ;
#5669=CARTESIAN_POINT ( 'NONE',  ( -30.98076211353325249, 14.99999999999984190, -2.500000000000000000 ) ) ;
#5679=DIRECTION ( 'NONE',  ( 1.000000000000000000, -0.000000000000000000, -0.000000000000000000 ) ) ;
#5694=EDGE_LOOP ( 'NONE', ( #4363, #4052, #887, #863 ) ) ;
#5696=CARTESIAN_POINT ( 'NONE',  ( 20.05579831881754060, 20.86490736922957367, 2.500000000000000444 ) ) ;
#5709=EDGE_CURVE ( 'NONE', #1228, #2958, #9698, .T. ) ;
#5721=VERTEX_POINT ( 'NONE', #7296 ) ;
#5726=EDGE_CURVE ( 'NONE', #4515, #8667, #1552, .T. ) ;
#5734=EDGE_CURVE ( 'NONE', #7593, #2609, #8235, .T. ) ;
#5735=EDGE_CURVE ( 'NONE', #4007, #670, #833, .T. ) ;
#5752=DIRECTION ( 'NONE',  ( -0.000000000000000000, -0.000000000000000000, -1.000000000000000000 ) ) ;
#5753=ORIENTED_EDGE ( 'NONE', *, *, #10128, .F. ) ;
#5755=CIRCLE ( 'NONE', #599, 4.500000000000000000 ) ;
#5765=CARTESIAN_POINT ( 'NONE',  ( 34.89248166448386002, 2.744837293030728098, 3.511881795860531952 ) ) ;
#5772=ORIENTED_EDGE ( 'NONE', *, *, #2167, .T. ) ;
#5779=AXIS2_PLACEMENT_3D ( 'NONE', #3244, #10972, #906 ) ;
#5781=DIRECTION ( 'NONE',  ( -1.000000000000000000, -6.098637220230964906E-17, -0.000000000000000000 ) ) ;
#5815=ADVANCED_FACE ( 'NONE', ( #7405 ), #2407, .T. ) ;
#5818=VECTOR ( 'NONE', #9885, 1000.000000000000000 ) ;
#5820=AXIS2_PLACEMENT_3D ( 'NONE', #1372, #10861, #3251 ) ;
#5825=ORIENTED_EDGE ( 'NONE', *, *, #4585, .F. ) ;
#5847=DIRECTION ( 'NONE',  ( 0.000000000000000000, 0.000000000000000000, 1.000000000000000000 ) ) ;
#5853=DIRECTION ( 'NONE',  ( -1.000000000000000000, -6.098637220230964906E-17, 0.000000000000000000 ) ) ;
#5864=ADVANCED_FACE ( 'NONE', ( #10079 ), #2470, .F. ) ;
#5876=EDGE_CURVE ( 'NONE', #3723, #4583, #9717, .T. ) ;
#5881=ORIENTED_EDGE ( 'NONE', *, *, #6656, .F. ) ;
#5927=EDGE_LOOP ( 'NONE', ( #4950, #10052, #6499, #1671 ) ) ;
#5931=ORIENTED_EDGE ( 'NONE', *, *, #3771, .T. ) ;
#5932=PLANE ( 'NONE',  #3970 ) ;
#5937=ORIENTED_EDGE ( 'NONE', *, *, #9425, .F. ) ;
#5939=CARTESIAN_POINT ( 'NONE',  ( 29.49999999999999645, -17.99999999999998579, 7.500000000000053291 ) ) ;
#5942=CIRCLE ( 'NONE', #7542, 2.649999999999992362 ) ;
#5948=CYLINDRICAL_SURFACE ( 'NONE', #6305, 24.99999999999999645 ) ;
#5949=ORIENTED_EDGE ( 'NONE', *, *, #2900, .T. ) ;
#5952=AXIS2_PLACEMENT_3D ( 'NONE', #9738, #5303, #447 ) ;
#5963=CARTESIAN_POINT ( 'NONE',  ( 34.99999999999999289, -3.999999999999993339, -4.999999999999995559 ) ) ;
#5997=CARTESIAN_POINT ( 'NONE',  ( 29.49999999999999289, 2.000000000000001776, -2.500000000000000000 ) ) ;
#6005=CARTESIAN_POINT ( 'NONE',  ( 29.49999999999999645, -3.999999999999993339, -4.999999999999995559 ) ) ;
#6019=PLANE ( 'NONE',  #1147 ) ;
#6021=EDGE_CURVE ( 'NONE', #6545, #3095, #6875, .T. ) ;
#6025=DIRECTION ( 'NONE',  ( -1.000000000000000000, 0.000000000000000000, 0.000000000000000000 ) ) ;
#6027=CARTESIAN_POINT ( 'NONE',  ( 34.80704760714189661, 3.674543421742908045, -2.801642449272108149 ) ) ;
#6042=ORIENTED_EDGE ( 'NONE', *, *, #8615, .T. ) ;
#6080=FACE_BOUND ( 'NONE', #2320, .T. ) ;
#6099=EDGE_CURVE ( 'NONE', #6333, #5356, #4634, .T. ) ;
#6111=CIRCLE ( 'NONE', #7175, 4.999999999999997335 ) ;
#6119=VECTOR ( 'NONE', #9946, 1000.000000000000000 ) ;
#6132=DIRECTION ( 'NONE',  ( 0.000000000000000000, 0.000000000000000000, 1.000000000000000000 ) ) ;
#6139=ORIENTED_EDGE ( 'NONE', *, *, #10269, .F. ) ;
#6140=FILL_AREA_STYLE ('',( #8320 ) ) ;
#6145=CARTESIAN_POINT ( 'NONE',  ( 29.49999999999999645, -9.999999999999998224, -10.50000000000000355 ) ) ;
#6161=AXIS2_PLACEMENT_3D ( 'NONE', #4810, #8188, #564 ) ;
#6186=VERTEX_POINT ( 'NONE', #9789 ) ;
#6188=CARTESIAN_POINT ( 'NONE',  ( 34.94281041931228771, 2.000000000000002220, 2.500000000000000000 ) ) ;
#6189=EDGE_CURVE ( 'NONE', #6838, #652, #7068, .T. ) ;
#6191=CARTESIAN_POINT ( 'NONE',  ( -21.21106610644865498, 16.50000000000026290, -9.500000000000000000 ) ) ;
#6203=EDGE_CURVE ( 'NONE', #609, #3529, #7126, .T. ) ;
#6205=CARTESIAN_POINT ( 'NONE',  ( 29.49999999999999289, -9.999999999999998224, 15.50000000000000711 ) ) ;
#6210=ADVANCED_FACE ( 'NONE', ( #448, #3848 ), #7233, .T. ) ;
#6222=CARTESIAN_POINT ( 'NONE',  ( 29.49999999999999289, 14.99999999999984546, 2.500000000000000000 ) ) ;
#6223=ORIENTED_EDGE ( 'NONE', *, *, #5550, .F. ) ;
#6230=VECTOR ( 'NONE', #8027, 1000.000000000000000 ) ;
#6235=ORIENTED_EDGE ( 'NONE', *, *, #5214, .T. ) ;
#6240=LINE ( 'NONE', #348, #674 ) ;
#6242=DIRECTION ( 'NONE',  ( -1.000000000000000000, -6.098637220230964906E-17, 0.000000000000000000 ) ) ;
#6249=VECTOR ( 'NONE', #10266, 1000.000000000000000 ) ;
#6256=DIRECTION ( 'NONE',  ( 0.000000000000000000, 0.000000000000000000, -1.000000000000000000 ) ) ;
#6259=CARTESIAN_POINT ( 'NONE',  ( -25.98076211353324894, 13.49999999999941913, -5.000000000000000000 ) ) ;
#6267=ORIENTED_EDGE ( 'NONE', *, *, #8656, .F. ) ;
#6268=EDGE_CURVE ( 'NONE', #3160, #5721, #2390, .T. ) ;
#6278=CARTESIAN_POINT ( 'NONE',  ( -2.649999999999991029, 30.00000000000000000, 2.500000000000000000 ) ) ;
#6294=CYLINDRICAL_SURFACE ( 'NONE', #10627, 4.500000000000000000 ) ;
#6296=DIRECTION ( 'NONE',  ( -0.000000000000000000, -0.000000000000000000, -1.000000000000000000 ) ) ;
#6305=AXIS2_PLACEMENT_3D ( 'NONE', #9338, #8619, #828 ) ;
#6306=VECTOR ( 'NONE', #398, 999.9999999999998863 ) ;
#6311=CARTESIAN_POINT ( 'NONE',  ( 34.99999999999999289, -3.999999999999993339, -7.149999999999983480 ) ) ;
#6324=CARTESIAN_POINT ( 'NONE',  ( 29.49999999999999289, 5.000000000000000888, 5.500000000000000000 ) ) ;
#6333=VERTEX_POINT ( 'NONE', #7334 ) ;
#6336=PRODUCT_DEFINITION_FORMATION_WITH_SPECIFIED_SOURCE ( 'ANY', '', #3417, .NOT_KNOWN. ) ;
#6345=DIRECTION ( 'NONE',  ( -1.000000000000000000, -6.098637220230964906E-17, 0.000000000000000000 ) ) ;
#6348=ORIENTED_EDGE ( 'NONE', *, *, #2201, .T. ) ;
#6357=FACE_OUTER_BOUND ( 'NONE', #4935, .T. ) ;
#6362=CARTESIAN_POINT ( 'NONE',  ( -5.076455387921347651, 24.47916666666666075, 2.499999999999999112 ) ) ;
#6365=ORIENTED_EDGE ( 'NONE', *, *, #1059, .F. ) ;
#6386=CARTESIAN_POINT ( 'NONE',  ( 34.74418829745650328, 4.228279689541292186, 2.594445730714923126 ) ) ;
#6391=EDGE_LOOP ( 'NONE', ( #7884, #4889, #5397, #3631, #1317, #1545, #5949, #2837, #10412, #10819, #7270, #334, #577, #10739 ) ) ;
#6406=DIRECTION ( 'NONE',  ( -4.312387734421983138E-17, 0.7071067811865463515, 0.7071067811865487940 ) ) ;
#6430=CARTESIAN_POINT ( 'NONE',  ( 34.86952523334974785, 3.022518564432433497, 3.235504471074991617 ) ) ;
#6461=VECTOR ( 'NONE', #6851, 1000.000000000000000 ) ;
#6463=CARTESIAN_POINT ( 'NONE',  ( 29.49999999999999645, 1.387778780781445676E-14, -12.49999999999999822 ) ) ;
#6467=PLANE ( 'NONE',  #9144 ) ;
#6470=CARTESIAN_POINT ( 'NONE',  ( 6.015568632492056977, 34.47916666666665009, -2.499999999999998668 ) ) ;
#6473=VECTOR ( 'NONE', #2746, 1000.000000000000000 ) ;
#6484=CARTESIAN_POINT ( 'NONE',  ( 34.93845944406324122, 2.080102445711406123, 4.707808283735069210 ) ) ;
#6486=VERTEX_POINT ( 'NONE', #10339 ) ;
#6497=CARTESIAN_POINT ( 'NONE',  ( 0.000000000000000000, 30.00000000000000000, 2.500000000000000000 ) ) ;
#6499=ORIENTED_EDGE ( 'NONE', *, *, #9675, .F. ) ;
#6516=EDGE_CURVE ( 'NONE', #3385, #7860, #1733, .T. ) ;
#6525=ORIENTED_EDGE ( 'NONE', *, *, #253, .F. ) ;
#6545=VERTEX_POINT ( 'NONE', #7065 ) ;
#6546=CARTESIAN_POINT ( 'NONE',  ( -21.21106610644865498, 13.49999999999941913, -5.000000000000000000 ) ) ;
#6558=ORIENTED_EDGE ( 'NONE', *, *, #457, .T. ) ;
#6560=LINE ( 'NONE', #9850, #2053 ) ;
#6567=EDGE_LOOP ( 'NONE', ( #2107, #7052, #3889, #10166, #10507 ) ) ;
#6569=CARTESIAN_POINT ( 'NONE',  ( 34.99999999999999289, -9.999999999999998224, -12.49999999999999822 ) ) ;
#6585=CARTESIAN_POINT ( 'NONE',  ( 34.82458596820516306, 3.503579405888650466, 2.892497030208068143 ) ) ;
#6589=ORIENTED_EDGE ( 'NONE', *, *, #603, .F. ) ;
#6590=CARTESIAN_POINT ( 'NONE',  ( 25.58039891549807976, 2.000000000000001776, -2.500000000000000444 ) ) ;
#6617=AXIS2_PLACEMENT_3D ( 'NONE', #6005, #1670, #1789 ) ;
#6623=DIRECTION ( 'NONE',  ( -0.000000000000000000, -0.000000000000000000, -1.000000000000000000 ) ) ;
#6626=EDGE_CURVE ( 'NONE', #4583, #3723, #2639, .T. ) ;
#6632=CARTESIAN_POINT ( 'NONE',  ( -30.75045812061784289, 13.49999999999941913, -9.500000000000000000 ) ) ;
#6635=DIRECTION ( 'NONE',  ( -0.000000000000000000, -1.000000000000000000, -0.000000000000000000 ) ) ;
#6647=CARTESIAN_POINT ( 'NONE',  ( -25.98076211353324894, 4.999999999999997335, 5.500000000000000000 ) ) ;
#6648=ORIENTED_EDGE ( 'NONE', *, *, #9460, .F. ) ;
#6652=ORIENTED_EDGE ( 'NONE', *, *, #7454, .T. ) ;
#6656=EDGE_CURVE ( 'NONE', #2434, #1386, #5342, .T. ) ;
#6662=VECTOR ( 'NONE', #3634, 1000.000000000000000 ) ;
#6669=ORIENTED_EDGE ( 'NONE', *, *, #5734, .F. ) ;
#6670=EDGE_CURVE ( 'NONE', #7102, #7683, #2793, .T. ) ;
#6680=PLANE ( 'NONE',  #8243 ) ;
#6688=CARTESIAN_POINT ( 'NONE',  ( 34.69578914996071717, 4.608685395970378629, -2.519144107514305730 ) ) ;
#6689=CARTESIAN_POINT ( 'NONE',  ( 34.99999999999999289, -3.999999999999993339, 7.850000000000012967 ) ) ;
#6690=ADVANCED_FACE ( 'NONE', ( #7953 ), #7846, .T. ) ;
#6692=DIRECTION ( 'NONE',  ( -1.000000000000000000, 0.000000000000000000, 0.000000000000000000 ) ) ;
#6694=B_SPLINE_CURVE_WITH_KNOTS ( 'NONE', 3,
 ( #10766, #10664, #5667, #6386, #3106, #10821, #6585, #3008, #6430, #5765, #7217, #9829, #2275, #6484, #7321, #1389 ),
 .UNSPECIFIED., .F., .F.,
 ( 4, 2, 2, 2, 2, 2, 2, 4 ),
 ( 0.000000000000000000, 0.0005875779155018993763, 0.001175155831003798753, 0.001762733746505697804, 0.002350311662007597505, 0.002937889577509496773, 0.003525467493011394740, 0.004700623324015191541 ),
 .UNSPECIFIED. ) ;
#6703=VECTOR ( 'NONE', #6709, 1000.000000000000000 ) ;
#6705=AXIS2_PLACEMENT_3D ( 'NONE', #1643, #6802, #5038 ) ;
#6706=DIRECTION ( 'NONE',  ( 1.000000000000000000, -0.000000000000000000, -0.000000000000000000 ) ) ;
#6709=DIRECTION ( 'NONE',  ( -0.000000000000000000, -0.000000000000000000, 1.000000000000000000 ) ) ;
#6713=CARTESIAN_POINT ( 'NONE',  ( 34.94281041931228771, 2.000000000000002220, -5.500000000000000000 ) ) ;
#6716=DIRECTION ( 'NONE',  ( -0.000000000000000000, -0.000000000000000000, -1.000000000000000000 ) ) ;
#6723=CYLINDRICAL_SURFACE ( 'NONE', #8141, 34.99999999999999289 ) ;
#6730=EDGE_LOOP ( 'NONE', ( #5937, #9639, #1040, #9613 ) ) ;
#6741=DIRECTION ( 'NONE',  ( -1.000000000000000000, 0.000000000000000000, 0.000000000000000000 ) ) ;
#6751=LINE ( 'NONE', #3643, #4554 ) ;
#6752=ORIENTED_EDGE ( 'NONE', *, *, #9498, .T. ) ;
#6753=DIRECTION ( 'NONE',  ( 0.000000000000000000, 0.000000000000000000, 1.000000000000000000 ) ) ;
#6758=LINE ( 'NONE', #1882, #6249 ) ;
#6763=CYLINDRICAL_SURFACE ( 'NONE', #5046, 2.149999999999988809 ) ;
#6770=CARTESIAN_POINT ( 'NONE',  ( 24.30992024302469900, 5.833333333333329485, -2.500000000000000000 ) ) ;
#6774=EDGE_CURVE ( 'NONE', #10496, #5165, #3010, .T. ) ;
#6778=VERTEX_POINT ( 'NONE', #5669 ) ;
#6781=ORIENTED_EDGE ( 'NONE', *, *, #2738, .F. ) ;
#6783=AXIS2_PLACEMENT_3D ( 'NONE', #2607, #3492, #10208 ) ;
#6784=ORIENTED_EDGE ( 'NONE', *, *, #6189, .F. ) ;
#6795=ADVANCED_BREP_SHAPE_REPRESENTATION ( '', ( #5559, #308 ), #5109 ) ;
#6800=DIRECTION ( 'NONE',  ( 0.000000000000000000, 0.000000000000000000, 1.000000000000000000 ) ) ;
#6802=DIRECTION ( 'NONE',  ( -0.000000000000000000, -0.000000000000000000, -1.000000000000000000 ) ) ;
#6823=ORIENTED_EDGE ( 'NONE', *, *, #3987, .F. ) ;
#6825=DIRECTION ( 'NONE',  ( -0.000000000000000000, -0.000000000000000000, -1.000000000000000000 ) ) ;
#6838=VERTEX_POINT ( 'NONE', #4835 ) ;
#6840=VERTEX_POINT ( 'NONE', #8211 ) ;
#6851=DIRECTION ( 'NONE',  ( -0.000000000000000000, 1.000000000000000000, -0.000000000000000000 ) ) ;
#6853=VERTEX_POINT ( 'NONE', #4051 ) ;
#6856=DIRECTION ( 'NONE',  ( 0.000000000000000000, 0.000000000000000000, -1.000000000000000000 ) ) ;
#6859=CARTESIAN_POINT ( 'NONE',  ( 34.85635190221861990, 3.172051726186627008, -3.113055717248542464 ) ) ;
#6865=DIRECTION ( 'NONE',  ( 0.000000000000000000, 0.000000000000000000, 1.000000000000000000 ) ) ;
#6875=CIRCLE ( 'NONE', #2095, 4.999999999999997335 ) ;
#6881=FACE_OUTER_BOUND ( 'NONE', #6730, .T. ) ;
#6887=VECTOR ( 'NONE', #10395, 1000.000000000000000 ) ;
#6890=LINE ( 'NONE', #162, #2046 ) ;
#6896=ADVANCED_FACE ( 'NONE', ( #9888, #2278, #10994 ), #5932, .F. ) ;
#6911=DIRECTION ( 'NONE',  ( 0.000000000000000000, 0.000000000000000000, 1.000000000000000000 ) ) ;
#6915=VERTEX_POINT ( 'NONE', #4275 ) ;
#6925=ADVANCED_FACE ( 'NONE', ( #1716 ), #3264, .F. ) ;
#6926=VERTEX_POINT ( 'NONE', #6713 ) ;
#6933=DIRECTION ( 'NONE',  ( 1.000000000000000000, -0.000000000000000000, -0.000000000000000000 ) ) ;
#6939=ORIENTED_EDGE ( 'NONE', *, *, #9838, .T. ) ;
#6952=VERTEX_POINT ( 'NONE', #39 ) ;
#6956=CARTESIAN_POINT ( 'NONE',  ( 0.000000000000000000, 0.000000000000000000, 0.000000000000000000 ) ) ;
#6958=CARTESIAN_POINT ( 'NONE',  ( 34.99999999999999289, -3.999999999999993339, -4.999999999999995559 ) ) ;
#6968=EDGE_CURVE ( 'NONE', #6545, #6778, #8602, .T. ) ;
#6972=CYLINDRICAL_SURFACE ( 'NONE', #5433, 7.500000000000000000 ) ;
#6975=ADVANCED_FACE ( 'NONE', ( #6881 ), #10051, .F. ) ;
#7002=CARTESIAN_POINT ( 'NONE',  ( 34.99999999999999289, -3.999999999999993339, -2.850000000000008082 ) ) ;
#7005=ORIENTED_EDGE ( 'NONE', *, *, #5734, .T. ) ;
#7008=VERTEX_POINT ( 'NONE', #2438 ) ;
#7009=ADVANCED_FACE ( 'NONE', ( #4392 ), #6763, .F. ) ;
#7012=AXIS2_PLACEMENT_3D ( 'NONE', #3099, #10040, #4827 ) ;
#7037=CARTESIAN_POINT ( 'NONE',  ( 29.49999999999999289, 6.938893903907228378E-15, 17.50000000000000000 ) ) ;
#7040=( LENGTH_UNIT ( ) NAMED_UNIT ( * ) SI_UNIT ( .MILLI., .METRE. ) );
#7045=DIRECTION ( 'NONE',  ( -0.000000000000000000, 1.000000000000000000, -0.000000000000000000 ) ) ;
#7052=ORIENTED_EDGE ( 'NONE', *, *, #3291, .F. ) ;
#7058=CARTESIAN_POINT ( 'NONE',  ( -25.98076211353324894, 14.99999999999984190, -2.500000000000000000 ) ) ;
#7059=AXIS2_PLACEMENT_3D ( 'NONE', #1982, #4541, #2302 ) ;
#7064=EDGE_LOOP ( 'NONE', ( #2737, #3462, #8468, #2974 ) ) ;
#7065=CARTESIAN_POINT ( 'NONE',  ( -30.98076211353325249, 14.99999999999984190, 2.500000000000000000 ) ) ;
#7068=CIRCLE ( 'NONE', #2271, 2.149999999999987921 ) ;
#7082=FACE_OUTER_BOUND ( 'NONE', #8394, .T. ) ;
#7091=CARTESIAN_POINT ( 'NONE',  ( 34.99999999999999289, 2.000000000000002220, -12.49999999999999822 ) ) ;
#7100=LINE ( 'NONE', #8041, #10857 ) ;
#7102=VERTEX_POINT ( 'NONE', #812 ) ;
#7105=LINE ( 'NONE', #2049, #9839 ) ;
#7123=CIRCLE ( 'NONE', #10843, 7.500000000000000000 ) ;
#7126=LINE ( 'NONE', #9572, #10260 ) ;
#7138=ORIENTED_EDGE ( 'NONE', *, *, #8318, .T. ) ;
#7154=CARTESIAN_POINT ( 'NONE',  ( 29.49999999999999645, 1.000000000000004441, -11.50000000000000533 ) ) ;
#7158=DIRECTION ( 'NONE',  ( 1.156482317317871478E-16, -0.000000000000000000, -1.000000000000000000 ) ) ;
#7175=AXIS2_PLACEMENT_3D ( 'NONE', #346, #238, #2866 ) ;
#7191=EDGE_CURVE ( 'NONE', #8667, #4515, #8769, .T. ) ;
#7195=FACE_OUTER_BOUND ( 'NONE', #6391, .T. ) ;
#7199=VECTOR ( 'NONE', #6406, 1000.000000000000000 ) ;
#7207=ORIENTED_EDGE ( 'NONE', *, *, #236, .F. ) ;
#7209=APPLICATION_CONTEXT ( 'automotive_design' ) ;
#7210=PRODUCT_CONTEXT ( 'NONE', #4382, 'mechanical' ) ;
#7212=FACE_OUTER_BOUND ( 'NONE', #3023, .T. ) ;
#7213=AXIS2_PLACEMENT_3D ( 'NONE', #5360, #8741, #10580 ) ;
#7217=CARTESIAN_POINT ( 'NONE',  ( 34.90196196521935690, 2.620161469061431436, 3.662783066803843468 ) ) ;
#7228=EDGE_CURVE ( 'NONE', #670, #2953, #2030, .T. ) ;
#7233=PLANE ( 'NONE',  #3690 ) ;
#7246=EDGE_LOOP ( 'NONE', ( #3674, #2395, #7207, #4173, #9211, #6939, #7968, #667 ) ) ;
#7247=DIRECTION ( 'NONE',  ( -1.156482317317871725E-16, 0.000000000000000000, 1.000000000000000000 ) ) ;
#7255=DIRECTION ( 'NONE',  ( 0.000000000000000000, 0.000000000000000000, -1.000000000000000000 ) ) ;
#7260=ORIENTED_EDGE ( 'NONE', *, *, #8339, .F. ) ;
#7270=ORIENTED_EDGE ( 'NONE', *, *, #10301, .T. ) ;
#7275=ORIENTED_EDGE ( 'NONE', *, *, #8526, .F. ) ;
#7283=ORIENTED_EDGE ( 'NONE', *, *, #6203, .T. ) ;
#7290=CARTESIAN_POINT ( 'NONE',  ( 6.015568632492056977, 34.47916666666665009, 0.000000000000000000 ) ) ;
#7295=DIRECTION ( 'NONE',  ( -6.098637220230964906E-17, 1.000000000000000000, 0.000000000000000000 ) ) ;
#7296=CARTESIAN_POINT ( 'NONE',  ( 29.49999999999999289, 5.000000000000002665, -2.500000000000000000 ) ) ;
#7299=AXIS2_PLACEMENT_3D ( 'NONE', #3656, #6933, #6256 ) ;
#7307=LINE ( 'NONE', #7471, #8911 ) ;
#7321=CARTESIAN_POINT ( 'NONE',  ( 34.94281041931229481, 2.000000000000001332, 5.102623512424888652 ) ) ;
#7323=ORIENTED_EDGE ( 'NONE', *, *, #8938, .T. ) ;
#7333=CARTESIAN_POINT ( 'NONE',  ( 34.99999999999999289, -3.999999999999993339, 10.00000000000000533 ) ) ;
#7334=CARTESIAN_POINT ( 'NONE',  ( 2.649999999999991029, 30.00000000000000000, 2.500000000000000000 ) ) ;
#7337=ORIENTED_EDGE ( 'NONE', *, *, #7967, .F. ) ;
#7341=DIRECTION ( 'NONE',  ( 0.000000000000000000, -1.000000000000000000, 0.000000000000000000 ) ) ;
#7364=AXIS2_PLACEMENT_3D ( 'NONE', #7946, #1220, #2845 ) ;
#7368=CARTESIAN_POINT ( 'NONE',  ( -21.21106610644865498, 13.49999999999941913, -2.500000000000000000 ) ) ;
#7405=FACE_OUTER_BOUND ( 'NONE', #6567, .T. ) ;
#7435=ADVANCED_FACE ( 'NONE', ( #9251 ), #4205, .F. ) ;
#7454=EDGE_CURVE ( 'NONE', #8327, #670, #84, .T. ) ;
#7460=CARTESIAN_POINT ( 'NONE',  ( -30.75045812061784289, 13.49999999999941913, -2.500000000000000000 ) ) ;
#7466=DIRECTION ( 'NONE',  ( -1.000000000000000000, -6.098637220230963674E-17, -1.156482317317871725E-16 ) ) ;
#7471=CARTESIAN_POINT ( 'NONE',  ( -30.31088913245546124, 17.49999999999980815, 2.500000000000000000 ) ) ;
#7486=EDGE_CURVE ( 'NONE', #6840, #10326, #10097, .T. ) ;
#7487=ORIENTED_EDGE ( 'NONE', *, *, #457, .F. ) ;
#7488=VERTEX_POINT ( 'NONE', #3314 ) ;
#7490=ORIENTED_EDGE ( 'NONE', *, *, #1729, .T. ) ;
#7499=EDGE_CURVE ( 'NONE', #4305, #8252, #4265, .T. ) ;
#7504=VERTEX_POINT ( 'NONE', #4320 ) ;
#7518=EDGE_LOOP ( 'NONE', ( #6784, #3288 ) ) ;
#7522=CARTESIAN_POINT ( 'NONE',  ( 34.86967549602668015, 3.020777328503463366, -3.237032597732066641 ) ) ;
#7523=DIRECTION ( 'NONE',  ( 6.098637220230963674E-17, -1.000000000000000000, 0.000000000000000000 ) ) ;
#7542=AXIS2_PLACEMENT_3D ( 'NONE', #7835, #2784, #5121 ) ;
#7544=PRESENTATION_STYLE_ASSIGNMENT (( #7763 ) ) ;
#7549=DIRECTION ( 'NONE',  ( -0.000000000000000000, -0.000000000000000000, -1.000000000000000000 ) ) ;
#7552=EDGE_LOOP ( 'NONE', ( #5825, #6589 ) ) ;
#7561=CYLINDRICAL_SURFACE ( 'NONE', #4290, 4.999999999999997335 ) ;
#7562=EDGE_LOOP ( 'NONE', ( #6648, #809, #3388, #3207, #2942, #8280, #768, #2123 ) ) ;
#7565=ORIENTED_EDGE ( 'NONE', *, *, #9663, .F. ) ;
#7575=CARTESIAN_POINT ( 'NONE',  ( 34.99999999999999289, -3.999999999999993339, 12.14999999999999680 ) ) ;
#7583=AXIS2_PLACEMENT_3D ( 'NONE', #4647, #8032, #7247 ) ;
#7593=VERTEX_POINT ( 'NONE', #6546 ) ;
#7622=ORIENTED_EDGE ( 'NONE', *, *, #1271, .T. ) ;
#7630=CARTESIAN_POINT ( 'NONE',  ( -21.21106610644865498, 16.50000000000026290, -2.500000000000000000 ) ) ;
#7635=DIRECTION ( 'NONE',  ( 0.000000000000000000, 0.000000000000000000, 1.000000000000000000 ) ) ;
#7651=CARTESIAN_POINT ( 'NONE',  ( 29.49999999999999645, 2.000000000000001776, -12.49999999999999822 ) ) ;
#7654=EDGE_CURVE ( 'NONE', #9249, #4777, #9049, .T. ) ;
#7662=VERTEX_POINT ( 'NONE', #1549 ) ;
#7663=DIRECTION ( 'NONE',  ( 0.000000000000000000, -0.000000000000000000, 1.000000000000000000 ) ) ;
#7665=CARTESIAN_POINT ( 'NONE',  ( 23.05579831881754416, 20.86490736922957367, 14.50000000000000000 ) ) ;
#7678=ORIENTED_EDGE ( 'NONE', *, *, #5726, .F. ) ;
#7681=ORIENTED_EDGE ( 'NONE', *, *, #6099, .T. ) ;
#7683=VERTEX_POINT ( 'NONE', #814 ) ;
#7686=( NAMED_UNIT ( * ) PLANE_ANGLE_UNIT ( ) SI_UNIT ( $, .RADIAN. ) );
#7692=CARTESIAN_POINT ( 'NONE',  ( -9.167668597118891028E-15, -10.00000000000000000, 15.49999999999998757 ) ) ;
#7698=CARTESIAN_POINT ( 'NONE',  ( 34.90224802882303834, 2.616310811731262120, -3.667896704194530511 ) ) ;
#7700=CARTESIAN_POINT ( 'NONE',  ( -25.98076211353324894, 4.999999999999997335, 2.500000000000000000 ) ) ;
#7707=ORIENTED_EDGE ( 'NONE', *, *, #6268, .T. ) ;
#7711=ADVANCED_FACE ( 'NONE', ( #4220 ), #5115, .F. ) ;
#7718=AXIS2_PLACEMENT_3D ( 'NONE', #2551, #7549, #8435 ) ;
#7719=VERTEX_POINT ( 'NONE', #7665 ) ;
#7720=DIRECTION ( 'NONE',  ( -0.000000000000000000, -0.000000000000000000, -1.000000000000000000 ) ) ;
#7725=DIRECTION ( 'NONE',  ( 0.000000000000000000, 0.000000000000000000, 1.000000000000000000 ) ) ;
#7742=SURFACE_STYLE_FILL_AREA ( #10238 ) ;
#7749=DIRECTION ( 'NONE',  ( 0.000000000000000000, 0.000000000000000000, -1.000000000000000000 ) ) ;
#7753=CARTESIAN_POINT ( 'NONE',  ( 29.17190429162963738, 6.999999999999999112, 2.500000000000000000 ) ) ;
#7755=CARTESIAN_POINT ( 'NONE',  ( 34.91794119163850496, 2.397787035234374198, -3.994322637888107597 ) ) ;
#7763=SURFACE_STYLE_USAGE ( .BOTH. , #1932 ) ;
#7781=DIRECTION ( 'NONE',  ( -1.000000000000000000, 0.000000000000000000, 0.000000000000000000 ) ) ;
#7783=ORIENTED_EDGE ( 'NONE', *, *, #9838, .F. ) ;
#7788=VECTOR ( 'NONE', #1359, 1000.000000000000000 ) ;
#7794=CARTESIAN_POINT ( 'NONE',  ( 29.49999999999999645, -3.999999999999993339, -2.850000000000008082 ) ) ;
#7797=ORIENTED_EDGE ( 'NONE', *, *, #555, .T. ) ;
#7800=VERTEX_POINT ( 'NONE', #3386 ) ;
#7810=ORIENTED_EDGE ( 'NONE', *, *, #4190, .F. ) ;
#7812=DIRECTION ( 'NONE',  ( 0.000000000000000000, 0.000000000000000000, 1.000000000000000000 ) ) ;
#7819=DIRECTION ( 'NONE',  ( 1.000000000000000000, 0.000000000000000000, 6.308085367188384325E-16 ) ) ;
#7821=ORIENTED_EDGE ( 'NONE', *, *, #4917, .T. ) ;
#7824=DIRECTION ( 'NONE',  ( 1.000000000000000000, -0.000000000000000000, -0.000000000000000000 ) ) ;
#7827=CARTESIAN_POINT ( 'NONE',  ( -21.65063509461104374, 12.49999999999986322, 2.500000000000000000 ) ) ;
#7835=CARTESIAN_POINT ( 'NONE',  ( 0.000000000000000000, 30.00000000000000000, -2.500000000000000000 ) ) ;
#7838=ADVANCED_FACE ( 'NONE', ( #1660 ), #9433, .T. ) ;
#7846=CYLINDRICAL_SURFACE ( 'NONE', #8295, 1.500000000000001332 ) ;
#7855=CARTESIAN_POINT ( 'NONE',  ( 2.649999999999992362, 30.00000000000000000, -2.500000000000000000 ) ) ;
#7858=DIRECTION ( 'NONE',  ( -0.000000000000000000, 0.000000000000000000, -1.000000000000000000 ) ) ;
#7860=VERTEX_POINT ( 'NONE', #10499 ) ;
#7866=CIRCLE ( 'NONE', #568, 34.99999999999999289 ) ;
#7884=ORIENTED_EDGE ( 'NONE', *, *, #3498, .F. ) ;
#7888=ORIENTED_EDGE ( 'NONE', *, *, #1594, .F. ) ;
#7906=AXIS2_PLACEMENT_3D ( 'NONE', #8478, #4437, #7819 ) ;
#7910=AXIS2_PLACEMENT_3D ( 'NONE', #8274, #3218, #9745 ) ;
#7920=VECTOR ( 'NONE', #7523, 1000.000000000000000 ) ;
#7926=DIRECTION ( 'NONE',  ( -0.000000000000000000, -0.000000000000000000, -1.000000000000000000 ) ) ;
#7928=DIRECTION ( 'NONE',  ( -0.000000000000000000, -0.000000000000000000, -1.000000000000000000 ) ) ;
#7930=PLANE ( 'NONE',  #2805 ) ;
#7932=CARTESIAN_POINT ( 'NONE',  ( -2.649999999999992362, 30.00000000000000000, -2.500000000000000000 ) ) ;
#7945=CARTESIAN_POINT ( 'NONE',  ( -25.98076211353324894, 16.50000000000026290, -5.000000000000000000 ) ) ;
#7946=CARTESIAN_POINT ( 'NONE',  ( 0.000000000000000000, 30.00000000000000000, -23.71320343559643007 ) ) ;
#7953=FACE_OUTER_BOUND ( 'NONE', #563, .T. ) ;
#7967=EDGE_CURVE ( 'NONE', #6486, #4305, #1949, .T. ) ;
#7968=ORIENTED_EDGE ( 'NONE', *, *, #1250, .T. ) ;
#7970=CARTESIAN_POINT ( 'NONE',  ( 29.49999999999999645, 1.387778780781445676E-14, -12.49999999999999822 ) ) ;
#7973=CYLINDRICAL_SURFACE ( 'NONE', #9325, 24.99999999999999645 ) ;
#7978=FACE_OUTER_BOUND ( 'NONE', #690, .T. ) ;
#7983=EDGE_CURVE ( 'NONE', #2134, #6926, #7105, .T. ) ;
#7992=DIRECTION ( 'NONE',  ( -1.000000000000000000, -6.098637220230964906E-17, -6.308085367188384325E-16 ) ) ;
#8002=CYLINDRICAL_SURFACE ( 'NONE', #1329, 2.149999999999990585 ) ;
#8018=FACE_OUTER_BOUND ( 'NONE', #8703, .T. ) ;
#8025=CARTESIAN_POINT ( 'NONE',  ( 34.99999999999999289, -2.999999999999977796, -17.49999999999999645 ) ) ;
#8027=DIRECTION ( 'NONE',  ( 0.000000000000000000, 0.000000000000000000, 1.000000000000000000 ) ) ;
#8032=DIRECTION ( 'NONE',  ( -1.000000000000000000, -6.098637220230963674E-17, -1.156482317317871725E-16 ) ) ;
#8038=DIRECTION ( 'NONE',  ( 0.000000000000000000, 0.000000000000000000, 1.000000000000000000 ) ) ;
#8041=CARTESIAN_POINT ( 'NONE',  ( 29.49999999999999289, 6.938893903907228378E-15, 17.50000000000000000 ) ) ;
#8045=EDGE_CURVE ( 'NONE', #1687, #7662, #10914, .T. ) ;
#8046=EDGE_LOOP ( 'NONE', ( #2322, #4101, #8956, #7138 ) ) ;
#8051=CARTESIAN_POINT ( 'NONE',  ( 0.000000000000000000, 0.000000000000000000, -2.500000000000000000 ) ) ;
#8052=ORIENTED_EDGE ( 'NONE', *, *, #9101, .T. ) ;
#8059=AXIS2_PLACEMENT_3D ( 'NONE', #6632, #10203, #5158 ) ;
#8063=VECTOR ( 'NONE', #7824, 1000.000000000000000 ) ;
#8066=EDGE_LOOP ( 'NONE', ( #2077, #10852, #10065, #5931, #551 ) ) ;
#8068=VECTOR ( 'NONE', #10547, 1000.000000000000000 ) ;
#8075=CIRCLE ( 'NONE', #10911, 2.149999999999992362 ) ;
#8085=DIRECTION ( 'NONE',  ( -6.098637220230963674E-17, 1.000000000000000000, 0.000000000000000000 ) ) ;
#8092=LINE ( 'NONE', #1201, #10563 ) ;
#8100=ORIENTED_EDGE ( 'NONE', *, *, #4180, .T. ) ;
#8102=CARTESIAN_POINT ( 'NONE',  ( 0.000000000000000000, 0.000000000000000000, 2.500000000000000000 ) ) ;
#8114=ORIENTED_EDGE ( 'NONE', *, *, #8045, .F. ) ;
#8130=AXIS2_PLACEMENT_3D ( 'NONE', #180, #6911, #5141 ) ;
#8141=AXIS2_PLACEMENT_3D ( 'NONE', #5639, #10116, #2503 ) ;
#8150=FACE_OUTER_BOUND ( 'NONE', #5694, .T. ) ;
#8156=PLANE ( 'NONE',  #7012 ) ;
#8170=ADVANCED_FACE ( 'NONE', ( #9302 ), #5097, .T. ) ;
#8173=LINE ( 'NONE', #1560, #5600 ) ;
#8175=ORIENTED_EDGE ( 'NONE', *, *, #573, .T. ) ;
#8176=ORIENTED_EDGE ( 'NONE', *, *, #4585, .T. ) ;
#8188=DIRECTION ( 'NONE',  ( 0.000000000000000000, 0.000000000000000000, 1.000000000000000000 ) ) ;
#8200=DIRECTION ( 'NONE',  ( -1.000000000000000000, 0.000000000000000000, 0.000000000000000000 ) ) ;
#8207=ORIENTED_EDGE ( 'NONE', *, *, #7654, .T. ) ;
#8208=DIRECTION ( 'NONE',  ( -1.000000000000000000, 0.000000000000000000, 0.000000000000000000 ) ) ;
#8211=CARTESIAN_POINT ( 'NONE',  ( -30.75045812061784289, 13.49999999999941913, -5.000000000000000000 ) ) ;
#8228=CARTESIAN_POINT ( 'NONE',  ( 29.49999999999999645, -2.999999999999978240, -17.49999999999999645 ) ) ;
#8235=LINE ( 'NONE', #9966, #3855 ) ;
#8237=ORIENTED_EDGE ( 'NONE', *, *, #1729, .F. ) ;
#8243=AXIS2_PLACEMENT_3D ( 'NONE', #3914, #7295, #9026 ) ;
#8246=CARTESIAN_POINT ( 'NONE',  ( 0.000000000000000000, 30.00000000000000000, -2.500000000000000000 ) ) ;
#8252=VERTEX_POINT ( 'NONE', #879 ) ;
#8263=ORIENTED_EDGE ( 'NONE', *, *, #1433, .T. ) ;
#8265=ORIENTED_EDGE ( 'NONE', *, *, #1622, .T. ) ;
#8266=EDGE_CURVE ( 'NONE', #1687, #7008, #6890, .T. ) ;
#8274=CARTESIAN_POINT ( 'NONE',  ( 29.49999999999999645, 1.387778780781445676E-14, -12.49999999999999822 ) ) ;
#8280=ORIENTED_EDGE ( 'NONE', *, *, #10269, .T. ) ;
#8286=CIRCLE ( 'NONE', #9895, 5.000000000000000888 ) ;
#8289=ADVANCED_FACE ( 'NONE', ( #1046 ), #9437, .F. ) ;
#8291=DIRECTION ( 'NONE',  ( -1.000000000000000000, -6.098637220230964906E-17, -6.308085367188384325E-16 ) ) ;
#8295=AXIS2_PLACEMENT_3D ( 'NONE', #9609, #10510, #3726 ) ;
#8299=LINE ( 'NONE', #6463, #8598 ) ;
#8317=ORIENTED_EDGE ( 'NONE', *, *, #1459, .F. ) ;
#8318=EDGE_CURVE ( 'NONE', #5165, #5356, #5942, .T. ) ;
#8320=FILL_AREA_STYLE_COLOUR ( '', #4771 ) ;
#8327=VERTEX_POINT ( 'NONE', #6770 ) ;
#8329=DIRECTION ( 'NONE',  ( 0.000000000000000000, 0.000000000000000000, 1.000000000000000000 ) ) ;
#8339=EDGE_CURVE ( 'NONE', #7488, #8693, #2554, .T. ) ;
#8341=EDGE_CURVE ( 'NONE', #5356, #5165, #4360, .T. ) ;
#8394=EDGE_LOOP ( 'NONE', ( #4734, #6267, #5522, #5306 ) ) ;
#8402=DIRECTION ( 'NONE',  ( -1.000000000000000000, 0.000000000000000000, 0.000000000000000000 ) ) ;
#8407=DIRECTION ( 'NONE',  ( 0.000000000000000000, 1.000000000000000000, 0.000000000000000000 ) ) ;
#8409=CARTESIAN_POINT ( 'NONE',  ( 34.64101615137754209, 5.000000000000001776, -2.500000000000000000 ) ) ;
#8418=VECTOR ( 'NONE', #10849, 1000.000000000000000 ) ;
#8422=LINE ( 'NONE', #1821, #1691 ) ;
#8432=EDGE_LOOP ( 'NONE', ( #2961, #4078, #7888, #2631 ) ) ;
#8435=DIRECTION ( 'NONE',  ( -1.000000000000000000, 0.000000000000000000, 0.000000000000000000 ) ) ;
#8450=CARTESIAN_POINT ( 'NONE',  ( -21.21106610644865498, 16.50000000000026290, -5.000000000000000000 ) ) ;
#8453=ORIENTED_EDGE ( 'NONE', *, *, #5493, .T. ) ;
#8459=LINE ( 'NONE', #7630, #2156 ) ;
#8468=ORIENTED_EDGE ( 'NONE', *, *, #7654, .F. ) ;
#8478=CARTESIAN_POINT ( 'NONE',  ( 29.49999999999999289, 2.000000000000001776, 17.50000000000000000 ) ) ;
#8479=DIRECTION ( 'NONE',  ( -1.000000000000000000, 0.000000000000000000, 0.000000000000000000 ) ) ;
#8485=CIRCLE ( 'NONE', #8130, 34.99999999999999289 ) ;
#8491=CARTESIAN_POINT ( 'NONE',  ( 34.99999999999999289, -3.999999999999993339, 10.00000000000000533 ) ) ;
#8496=ADVANCED_FACE ( 'NONE', ( #7212 ), #8002, .F. ) ;
#8507=ORIENTED_EDGE ( 'NONE', *, *, #20, .F. ) ;
#8526=EDGE_CURVE ( 'NONE', #6952, #1362, #8958, .T. ) ;
#8528=ADVANCED_FACE ( 'NONE', ( #4037 ), #8156, .F. ) ;
#8531=CARTESIAN_POINT ( 'NONE',  ( 34.94281041931228771, 2.000000000000002220, -5.500000000000000000 ) ) ;
#8551=ORIENTED_EDGE ( 'NONE', *, *, #8672, .F. ) ;
#8552=CARTESIAN_POINT ( 'NONE',  ( 20.05579831881754060, 20.86490736922957367, 14.50000000000000000 ) ) ;
#8573=DIRECTION ( 'NONE',  ( -0.000000000000000000, -0.000000000000000000, -1.000000000000000000 ) ) ;
#8582=DIRECTION ( 'NONE',  ( 0.000000000000000000, 0.000000000000000000, 1.000000000000000000 ) ) ;
#8589=( NAMED_UNIT ( * ) PLANE_ANGLE_UNIT ( ) SI_UNIT ( $, .RADIAN. ) );
#8593=VECTOR ( 'NONE', #6753, 1000.000000000000000 ) ;
#8598=VECTOR ( 'NONE', #3137, 1000.000000000000000 ) ;
#8602=LINE ( 'NONE', #4218, #3622 ) ;
#8611=AXIS2_PLACEMENT_3D ( 'NONE', #10131, #8573, #2518 ) ;
#8615=EDGE_CURVE ( 'NONE', #6840, #6853, #5755, .T. ) ;
#8619=DIRECTION ( 'NONE',  ( -0.000000000000000000, -0.000000000000000000, -1.000000000000000000 ) ) ;
#8632=LINE ( 'NONE', #4188, #6461 ) ;
#8641=CARTESIAN_POINT ( 'NONE',  ( 0.000000000000000000, 30.00000000000000000, 2.500000000000000000 ) ) ;
#8645=CARTESIAN_POINT ( 'NONE',  ( 29.49999999999999289, 14.99999999999984546, -2.500000000000000000 ) ) ;
#8656=EDGE_CURVE ( 'NONE', #2953, #4777, #9536, .T. ) ;
#8667=VERTEX_POINT ( 'NONE', #4547 ) ;
#8670=CARTESIAN_POINT ( 'NONE',  ( 5.076455387921339657, 24.47916666666667140, -2.499999999999998668 ) ) ;
#8672=EDGE_CURVE ( 'NONE', #6838, #10287, #8921, .T. ) ;
#8693=VERTEX_POINT ( 'NONE', #2038 ) ;
#8697=CARTESIAN_POINT ( 'NONE',  ( 0.000000000000000000, 30.00000000000000000, -23.71320343559643007 ) ) ;
#8703=EDGE_LOOP ( 'NONE', ( #8176, #6348, #6558, #10189 ) ) ;
#8716=VERTEX_POINT ( 'NONE', #6145 ) ;
#8727=ORIENTED_EDGE ( 'NONE', *, *, #8266, .F. ) ;
#8741=DIRECTION ( 'NONE',  ( 0.000000000000000000, 0.000000000000000000, 1.000000000000000000 ) ) ;
#8744=DIRECTION ( 'NONE',  ( -0.000000000000000000, -0.000000000000000000, -1.000000000000000000 ) ) ;
#8769=CIRCLE ( 'NONE', #3804, 2.149999999999990585 ) ;
#8771=DIRECTION ( 'NONE',  ( 0.000000000000000000, 8.673617379884032514E-16, 1.000000000000000000 ) ) ;
#8788=CIRCLE ( 'NONE', #4168, 2.149999999999988809 ) ;
#8792=LINE ( 'NONE', #3737, #269 ) ;
#8795=ORIENTED_EDGE ( 'NONE', *, *, #8990, .F. ) ;
#8803=DIRECTION ( 'NONE',  ( 1.000000000000000000, 0.000000000000000000, 0.000000000000000000 ) ) ;
#8813=FACE_BOUND ( 'NONE', #877, .T. ) ;
#8821=CARTESIAN_POINT ( 'NONE',  ( 5.076455387921339657, 24.47916666666667140, 2.500000000000000000 ) ) ;
#8832=ORIENTED_EDGE ( 'NONE', *, *, #1117, .F. ) ;
#8844=ORIENTED_EDGE ( 'NONE', *, *, #8938, .F. ) ;
#8855=DIRECTION ( 'NONE',  ( -0.000000000000000000, -0.000000000000000000, -1.000000000000000000 ) ) ;
#8865=CARTESIAN_POINT ( 'NONE',  ( 21.55579831881754416, 20.86490736922957367, 14.50000000000000000 ) ) ;
#8867=( NAMED_UNIT ( * ) PLANE_ANGLE_UNIT ( ) SI_UNIT ( $, .RADIAN. ) );
#8871=EDGE_CURVE ( 'NONE', #4305, #3617, #8299, .T. ) ;
#8886=DIRECTION ( 'NONE',  ( 0.000000000000000000, 0.000000000000000000, 1.000000000000000000 ) ) ;
#8896=EDGE_LOOP ( 'NONE', ( #7783, #6139, #10679, #2277 ) ) ;
#8903=CARTESIAN_POINT ( 'NONE',  ( 29.49999999999999645, -3.999999999999993339, -4.999999999999995559 ) ) ;
#8911=VECTOR ( 'NONE', #10808, 1000.000000000000000 ) ;
#8917=ORIENTED_EDGE ( 'NONE', *, *, #10884, .T. ) ;
#8921=LINE ( 'NONE', #6311, #8063 ) ;
#8923=EDGE_CURVE ( 'NONE', #6926, #3160, #2962, .T. ) ;
#8938=EDGE_CURVE ( 'NONE', #8693, #3385, #1638, .T. ) ;
#8941=VERTEX_POINT ( 'NONE', #2022 ) ;
#8956=ORIENTED_EDGE ( 'NONE', *, *, #6774, .T. ) ;
#8958=CIRCLE ( 'NONE', #5592, 34.99999999999999289 ) ;
#8959=ORIENTED_EDGE ( 'NONE', *, *, #1599, .T. ) ;
#8962=CARTESIAN_POINT ( 'NONE',  ( -9.899505063546603365E-15, 2.000000000000000000, 15.49999999999998046 ) ) ;
#8990=EDGE_CURVE ( 'NONE', #5059, #6778, #6111, .T. ) ;
#9001=ORIENTED_EDGE ( 'NONE', *, *, #3510, .F. ) ;
#9005=AXIS2_PLACEMENT_3D ( 'NONE', #4920, #680, #10905 ) ;
#9016=EDGE_LOOP ( 'NONE', ( #1283, #3002, #2696, #8551 ) ) ;
#9019=STYLED_ITEM ( 'NONE', ( #7544 ), #5559 ) ;
#9020=( GEOMETRIC_REPRESENTATION_CONTEXT ( 3 ) GLOBAL_UNCERTAINTY_ASSIGNED_CONTEXT ( ( #2591 ) ) GLOBAL_UNIT_ASSIGNED_CONTEXT ( ( #2637, #7686, #2740 ) ) REPRESENTATION_CONTEXT ( 'NONE', 'WORKASPACE' ) );
#9026=DIRECTION ( 'NONE',  ( -1.000000000000000000, -6.098637220230964906E-17, 0.000000000000000000 ) ) ;
#9028=ORIENTED_EDGE ( 'NONE', *, *, #7486, .F. ) ;
#9033=DIRECTION ( 'NONE',  ( 1.000000000000000000, -0.000000000000000000, -0.000000000000000000 ) ) ;
#9044=ORIENTED_EDGE ( 'NONE', *, *, #8871, .T. ) ;
#9049=LINE ( 'NONE', #6590, #2384 ) ;
#9050=ORIENTED_EDGE ( 'NONE', *, *, #2147, .T. ) ;
#9065=DIRECTION ( 'NONE',  ( 3.865177154556031370E-17, 0.7071067811865462405, -0.7071067811865489050 ) ) ;
#9069=CARTESIAN_POINT ( 'NONE',  ( -25.98076211353324894, 14.99999999999984190, -2.500000000000000000 ) ) ;
#9071=DIRECTION ( 'NONE',  ( -0.000000000000000000, -0.000000000000000000, -1.000000000000000000 ) ) ;
#9075=DIRECTION ( 'NONE',  ( 0.000000000000000000, 0.000000000000000000, 1.000000000000000000 ) ) ;
#9080=ADVANCED_FACE ( 'NONE', ( #4899 ), #1923, .F. ) ;
#9085=VECTOR ( 'NONE', #5325, 1000.000000000000000 ) ;
#9101=EDGE_CURVE ( 'NONE', #1491, #7008, #3980, .T. ) ;
#9115=DIRECTION ( 'NONE',  ( 1.000000000000000000, 6.098637220230964906E-17, 6.308085367188384325E-16 ) ) ;
#9121=ORIENTED_EDGE ( 'NONE', *, *, #9415, .F. ) ;
#9130=LINE ( 'NONE', #631, #7920 ) ;
#9144=AXIS2_PLACEMENT_3D ( 'NONE', #1263, #2937, #9868 ) ;
#9148=SURFACE_STYLE_FILL_AREA ( #6140 ) ;
#9152=ORIENTED_EDGE ( 'NONE', *, *, #3434, .T. ) ;
#9155=DIRECTION ( 'NONE',  ( -1.000000000000000000, 0.000000000000000000, 0.000000000000000000 ) ) ;
#9183=ORIENTED_EDGE ( 'NONE', *, *, #5876, .T. ) ;
#9185=MECHANICAL_DESIGN_GEOMETRIC_PRESENTATION_REPRESENTATION('',(#9360),#9020);
#9189=EDGE_CURVE ( 'NONE', #1386, #7504, #10777, .T. ) ;
#9211=ORIENTED_EDGE ( 'NONE', *, *, #5709, .T. ) ;
#9224=CARTESIAN_POINT ( 'NONE',  ( 29.49999999999999289, 5.000000000000001776, -2.500000000000000000 ) ) ;
#9227=VERTEX_POINT ( 'NONE', #46 ) ;
#9230=DIRECTION ( 'NONE',  ( 1.000000000000000000, 0.000000000000000000, 0.000000000000000000 ) ) ;
#9234=DIRECTION ( 'NONE',  ( 1.000000000000000000, 6.098637220230964906E-17, 6.308085367188384325E-16 ) ) ;
#9236=VERTEX_POINT ( 'NONE', #8670 ) ;
#9239=AXIS2_PLACEMENT_3D ( 'NONE', #9526, #2757, #6800 ) ;
#9241=CARTESIAN_POINT ( 'NONE',  ( 34.94170751511534689, 2.019541143081656998, -5.105981766738330485 ) ) ;
#9249=VERTEX_POINT ( 'NONE', #5997 ) ;
#9251=FACE_OUTER_BOUND ( 'NONE', #3229, .T. ) ;
#9260=EDGE_LOOP ( 'NONE', ( #2635, #8959 ) ) ;
#9302=FACE_OUTER_BOUND ( 'NONE', #1001, .T. ) ;
#9304=VERTEX_POINT ( 'NONE', #4398 ) ;
#9320=CARTESIAN_POINT ( 'NONE',  ( -25.98076211353324894, 14.99999999999984190, 2.500000000000000000 ) ) ;
#9325=AXIS2_PLACEMENT_3D ( 'NONE', #1246, #8744, #4588 ) ;
#9326=ORIENTED_EDGE ( 'NONE', *, *, #107, .F. ) ;
#9328=DIRECTION ( 'NONE',  ( -1.248995262339998101E-16, 0.7071067811865486830, 0.7071067811865463515 ) ) ;
#9329=VECTOR ( 'NONE', #5156, 1000.000000000000000 ) ;
#9338=CARTESIAN_POINT ( 'NONE',  ( 0.000000000000000000, 0.000000000000000000, 2.500000000000000000 ) ) ;
#9343=ORIENTED_EDGE ( 'NONE', *, *, #3291, .T. ) ;
#9345=SURFACE_STYLE_USAGE ( .BOTH. , #2572 ) ;
#9360=STYLED_ITEM ( 'NONE', ( #224 ), #6795 ) ;
#9367=FACE_OUTER_BOUND ( 'NONE', #8432, .T. ) ;
#9378=ORIENTED_EDGE ( 'NONE', *, *, #3422, .F. ) ;
#9394=EDGE_LOOP ( 'NONE', ( #10513, #8844, #7260, #10049 ) ) ;
#9404=FACE_OUTER_BOUND ( 'NONE', #9016, .T. ) ;
#9408=CARTESIAN_POINT ( 'NONE',  ( 21.55579831881754416, 20.86490736922957367, 14.50000000000000000 ) ) ;
#9411=CARTESIAN_POINT ( 'NONE',  ( 34.66939463810009414, 4.803388076618550606, -2.500000000000000888 ) ) ;
#9415=EDGE_CURVE ( 'NONE', #1215, #5059, #2044, .T. ) ;
#9416=CARTESIAN_POINT ( 'NONE',  ( -25.98076211353324894, 16.50000000000026290, -5.000000000000000000 ) ) ;
#9425=EDGE_CURVE ( 'NONE', #7800, #7683, #5415, .T. ) ;
#9427=AXIS2_PLACEMENT_3D ( 'NONE', #4288, #4170, #10286 ) ;
#9432=CARTESIAN_POINT ( 'NONE',  ( 25.58039891549807976, 2.000000000000001776, -12.50099999999999767 ) ) ;
#9433=CYLINDRICAL_SURFACE ( 'NONE', #3977, 34.99999999999999289 ) ;
#9437=CYLINDRICAL_SURFACE ( 'NONE', #1342, 2.149999999999990585 ) ;
#9443=DIRECTION ( 'NONE',  ( -0.000000000000000000, -0.000000000000000000, -1.000000000000000000 ) ) ;
#9444=ORIENTED_EDGE ( 'NONE', *, *, #4582, .T. ) ;
#9446=ADVANCED_FACE ( 'NONE', ( #9716 ), #374, .T. ) ;
#9457=LINE ( 'NONE', #4300, #1568 ) ;
#9460=EDGE_CURVE ( 'NONE', #2134, #6486, #5504, .T. ) ;
#9471=CARTESIAN_POINT ( 'NONE',  ( 29.49999999999999645, -7.999999999999996447, -12.49999999999999822 ) ) ;
#9479=EDGE_CURVE ( 'NONE', #234, #7800, #8422, .T. ) ;
#9495=CIRCLE ( 'NONE', #10027, 2.149999999999988809 ) ;
#9498=EDGE_CURVE ( 'NONE', #5409, #1804, #5269, .T. ) ;
#9502=DIRECTION ( 'NONE',  ( 0.000000000000000000, 0.000000000000000000, 1.000000000000000000 ) ) ;
#9512=CIRCLE ( 'NONE', #10752, 2.149999999999992362 ) ;
#9517=EDGE_LOOP ( 'NONE', ( #7678, #5233, #7490, #9326 ) ) ;
#9519=DIRECTION ( 'NONE',  ( 1.000000000000000000, 0.000000000000000000, -0.000000000000000000 ) ) ;
#9520=CIRCLE ( 'NONE', #7213, 7.500000000000000000 ) ;
#9526=CARTESIAN_POINT ( 'NONE',  ( 29.49999999999999645, 5.000000000000001776, -5.500000000000000000 ) ) ;
#9530=CARTESIAN_POINT ( 'NONE',  ( -21.65063509461104374, 12.49999999999986322, 2.500000000000000000 ) ) ;
#9536=LINE ( 'NONE', #4494, #10721 ) ;
#9543=VECTOR ( 'NONE', #7926, 1000.000000000000000 ) ;
#9546=ORIENTED_EDGE ( 'NONE', *, *, #5467, .T. ) ;
#9560=CARTESIAN_POINT ( 'NONE',  ( 21.55579831881754416, 20.86490736922957367, 2.500000000000000444 ) ) ;
#9565=DIRECTION ( 'NONE',  ( 1.000000000000000000, 0.000000000000000000, 0.000000000000000000 ) ) ;
#9572=CARTESIAN_POINT ( 'NONE',  ( -21.21106610644865498, 16.50000000000026290, -9.500000000000000000 ) ) ;
#9575=DIRECTION ( 'NONE',  ( -0.000000000000000000, -0.000000000000000000, -1.000000000000000000 ) ) ;
#9577=FACE_OUTER_BOUND ( 'NONE', #5513, .T. ) ;
#9579=CARTESIAN_POINT ( 'NONE',  ( 6.098637220230963427E-16, -10.00000000000000000, -10.50000000000000355 ) ) ;
#9597=ORIENTED_EDGE ( 'NONE', *, *, #5467, .F. ) ;
#9609=CARTESIAN_POINT ( 'NONE',  ( 21.55579831881754416, 20.86490736922957367, 14.50000000000000000 ) ) ;
#9613=ORIENTED_EDGE ( 'NONE', *, *, #2558, .F. ) ;
#9622=AXIS2_PLACEMENT_3D ( 'NONE', #2421, #10653, #3043 ) ;
#9639=ORIENTED_EDGE ( 'NONE', *, *, #793, .F. ) ;
#9646=FACE_OUTER_BOUND ( 'NONE', #9967, .T. ) ;
#9663=EDGE_CURVE ( 'NONE', #7719, #3723, #8092, .T. ) ;
#9674=DIRECTION ( 'NONE',  ( 1.000000000000000000, -0.000000000000000000, -0.000000000000000000 ) ) ;
#9675=EDGE_CURVE ( 'NONE', #7504, #7593, #10571, .T. ) ;
#9679=AXIS2_PLACEMENT_3D ( 'NONE', #468, #4655, #8038 ) ;
#9684=ORIENTED_EDGE ( 'NONE', *, *, #3358, .F. ) ;
#9698=LINE ( 'NONE', #7091, #2980 ) ;
#9716=FACE_OUTER_BOUND ( 'NONE', #3457, .T. ) ;
#9717=CIRCLE ( 'NONE', #6161, 1.500000000000001332 ) ;
#9736=VECTOR ( 'NONE', #616, 1000.000000000000000 ) ;
#9738=CARTESIAN_POINT ( 'NONE',  ( 34.99999999999999289, -3.999999999999993339, 10.00000000000000533 ) ) ;
#9745=DIRECTION ( 'NONE',  ( 1.000000000000000000, 6.098637220230964906E-17, 0.000000000000000000 ) ) ;
#9753=ORIENTED_EDGE ( 'NONE', *, *, #4921, .F. ) ;
#9754=FACE_BOUND ( 'NONE', #7552, .T. ) ;
#9761=EDGE_CURVE ( 'NONE', #4515, #590, #1939, .T. ) ;
#9776=ORIENTED_EDGE ( 'NONE', *, *, #9761, .F. ) ;
#9789=CARTESIAN_POINT ( 'NONE',  ( 34.99999999999999289, 7.372574772901430151E-15, 17.50000000000000355 ) ) ;
#9805=FACE_BOUND ( 'NONE', #4646, .T. ) ;
#9811=CARTESIAN_POINT ( 'NONE',  ( 34.99999999999999289, 16.00000000000000355, 1.499999999999947597 ) ) ;
#9821=ADVANCED_FACE ( 'NONE', ( #10805 ), #3919, .F. ) ;
#9822=EDGE_CURVE ( 'NONE', #3429, #8693, #9130, .T. ) ;
#9829=CARTESIAN_POINT ( 'NONE',  ( 34.91780110604603493, 2.399866884679865198, 3.990594396599065341 ) ) ;
#9838=EDGE_CURVE ( 'NONE', #2958, #6186, #2416, .T. ) ;
#9839=VECTOR ( 'NONE', #1995, 1000.000000000000000 ) ;
#9844=DIRECTION ( 'NONE',  ( 0.000000000000000000, 0.000000000000000000, -1.000000000000000000 ) ) ;
#9850=CARTESIAN_POINT ( 'NONE',  ( 29.49999999999999289, 16.00000000000000000, 1.499999999999945821 ) ) ;
#9851=AXIS2_PLACEMENT_3D ( 'NONE', #5963, #5143, #7749 ) ;
#9861=CARTESIAN_POINT ( 'NONE',  ( 6.098637220230963427E-16, -10.00000000000000000, 0.000000000000000000 ) ) ;
#9864=CIRCLE ( 'NONE', #1513, 4.999999999999997335 ) ;
#9865=DIRECTION ( 'NONE',  ( 0.000000000000000000, 0.000000000000000000, 1.000000000000000000 ) ) ;
#9868=DIRECTION ( 'NONE',  ( -1.000000000000000000, 0.000000000000000000, -0.000000000000000000 ) ) ;
#9885=DIRECTION ( 'NONE',  ( 1.156482317317871478E-16, -0.000000000000000000, -1.000000000000000000 ) ) ;
#9888=FACE_BOUND ( 'NONE', #317, .T. ) ;
#9895=AXIS2_PLACEMENT_3D ( 'NONE', #2087, #6296, #5364 ) ;
#9910=CIRCLE ( 'NONE', #10974, 2.149999999999992362 ) ;
#9919=LINE ( 'NONE', #6569, #10056 ) ;
#9946=DIRECTION ( 'NONE',  ( 0.000000000000000000, -1.000000000000000000, 0.000000000000000000 ) ) ;
#9960=LINE ( 'NONE', #8962, #10218 ) ;
#9966=CARTESIAN_POINT ( 'NONE',  ( -21.21106610644865498, 13.49999999999941913, -9.500000000000000000 ) ) ;
#9967=EDGE_LOOP ( 'NONE', ( #10665, #8265, #3261, #9044 ) ) ;
#9988=VERTEX_POINT ( 'NONE', #6689 ) ;
#9991=EDGE_LOOP ( 'NONE', ( #6235, #5262, #7275, #450, #7821, #10394 ) ) ;
#9993=ORIENTED_EDGE ( 'NONE', *, *, #20, .T. ) ;
#10004=ORIENTED_EDGE ( 'NONE', *, *, #2602, .T. ) ;
#10021=VERTEX_POINT ( 'NONE', #1300 ) ;
#10027=AXIS2_PLACEMENT_3D ( 'NONE', #2253, #7466, #9075 ) ;
#10040=DIRECTION ( 'NONE',  ( 0.000000000000000000, -0.000000000000000000, 1.000000000000000000 ) ) ;
#10049=ORIENTED_EDGE ( 'NONE', *, *, #1433, .F. ) ;
#10051=CYLINDRICAL_SURFACE ( 'NONE', #959, 2.999999999999999112 ) ;
#10052=ORIENTED_EDGE ( 'NONE', *, *, #2147, .F. ) ;
#10056=VECTOR ( 'NONE', #9865, 1000.000000000000000 ) ;
#10065=ORIENTED_EDGE ( 'NONE', *, *, #4190, .T. ) ;
#10069=ADVANCED_FACE ( 'NONE', ( #3745 ), #6972, .T. ) ;
#10079=FACE_OUTER_BOUND ( 'NONE', #753, .T. ) ;
#10094=ADVANCED_FACE ( 'NONE', ( #9577 ), #7973, .F. ) ;
#10097=LINE ( 'NONE', #5101, #420 ) ;
#10111=ORIENTED_EDGE ( 'NONE', *, *, #624, .F. ) ;
#10116=DIRECTION ( 'NONE',  ( -0.000000000000000000, -0.000000000000000000, -1.000000000000000000 ) ) ;
#10128=EDGE_CURVE ( 'NONE', #10904, #2973, #3588, .T. ) ;
#10131=CARTESIAN_POINT ( 'NONE',  ( 0.000000000000000000, 0.000000000000000000, -2.500000000000000000 ) ) ;
#10147=DIRECTION ( 'NONE',  ( 0.000000000000000000, 0.000000000000000000, 1.000000000000000000 ) ) ;
#10161=ORIENTED_EDGE ( 'NONE', *, *, #761, .F. ) ;
#10162=DIRECTION ( 'NONE',  ( 0.000000000000000000, 0.000000000000000000, -1.000000000000000000 ) ) ;
#10166=ORIENTED_EDGE ( 'NONE', *, *, #9415, .T. ) ;
#10189=ORIENTED_EDGE ( 'NONE', *, *, #2856, .F. ) ;
#10190=AXIS2_PLACEMENT_3D ( 'NONE', #1151, #4663, #157 ) ;
#10203=DIRECTION ( 'NONE',  ( 1.000000000000000000, -0.000000000000000000, 0.000000000000000000 ) ) ;
#10208=DIRECTION ( 'NONE',  ( 1.000000000000000000, 0.000000000000000000, 0.000000000000000000 ) ) ;
#10215=ORIENTED_EDGE ( 'NONE', *, *, #4312, .T. ) ;
#10218=VECTOR ( 'NONE', #9115, 1000.000000000000000 ) ;
#10221=CARTESIAN_POINT ( 'NONE',  ( -25.98076211353324894, 16.50000000000026290, -5.000000000000000000 ) ) ;
#10238=FILL_AREA_STYLE ('',( #119 ) ) ;
#10258=DIRECTION ( 'NONE',  ( -6.098637220230963674E-17, 1.000000000000000000, 0.000000000000000000 ) ) ;
#10259=ORIENTED_EDGE ( 'NONE', *, *, #8341, .T. ) ;
#10260=VECTOR ( 'NONE', #1294, 1000.000000000000000 ) ;
#10266=DIRECTION ( 'NONE',  ( 6.098637220230963674E-17, -1.000000000000000000, 0.000000000000000000 ) ) ;
#10269=EDGE_CURVE ( 'NONE', #234, #2958, #9960, .T. ) ;
#10275=ORIENTED_EDGE ( 'NONE', *, *, #2167, .F. ) ;
#10286=DIRECTION ( 'NONE',  ( 0.000000000000000000, 0.000000000000000000, 1.000000000000000000 ) ) ;
#10287=VERTEX_POINT ( 'NONE', #3906 ) ;
#10301=EDGE_CURVE ( 'NONE', #3429, #234, #6560, .T. ) ;
#10326=VERTEX_POINT ( 'NONE', #3234 ) ;
#10339=CARTESIAN_POINT ( 'NONE',  ( 29.49999999999999645, 2.000000000000001776, -10.50000000000000355 ) ) ;
#10350=CARTESIAN_POINT ( 'NONE',  ( -21.21106610644865498, 13.49999999999941913, -9.500000000000000000 ) ) ;
#10356=DIRECTION ( 'NONE',  ( -0.000000000000000000, -0.000000000000000000, -1.000000000000000000 ) ) ;
#10359=DIRECTION ( 'NONE',  ( 1.000000000000000000, 6.098637220230964906E-17, 6.308085367188384325E-16 ) ) ;
#10366=ORIENTED_EDGE ( 'NONE', *, *, #6021, .T. ) ;
#10384=AXIS2_PLACEMENT_3D ( 'NONE', #659, #8329, #2447 ) ;
#10386=CIRCLE ( 'NONE', #3284, 2.649999999999991029 ) ;
#10394=ORIENTED_EDGE ( 'NONE', *, *, #8923, .T. ) ;
#10395=DIRECTION ( 'NONE',  ( 1.000000000000000000, -0.000000000000000000, -0.000000000000000000 ) ) ;
#10406=DIRECTION ( 'NONE',  ( -0.000000000000000000, -1.000000000000000000, -0.000000000000000000 ) ) ;
#10412=ORIENTED_EDGE ( 'NONE', *, *, #8339, .T. ) ;
#10430=AXIS2_PLACEMENT_3D ( 'NONE', #6958, #9674, #2069 ) ;
#10447=CIRCLE ( 'NONE', #10617, 24.99999999999999645 ) ;
#10467=CARTESIAN_POINT ( 'NONE',  ( 29.49999999999999289, 2.000000000000001776, 15.49999999999999822 ) ) ;
#10480=CARTESIAN_POINT ( 'NONE',  ( -26.25045812061784289, 0.000000000000000000, -5.000000000000000000 ) ) ;
#10482=FACE_OUTER_BOUND ( 'NONE', #7246, .T. ) ;
#10496=VERTEX_POINT ( 'NONE', #6278 ) ;
#10499=CARTESIAN_POINT ( 'NONE',  ( 34.99999999999999289, -9.999999999999998224, 15.50000000000001243 ) ) ;
#10501=EDGE_LOOP ( 'NONE', ( #6781, #8052, #8727, #3049 ) ) ;
#10507=ORIENTED_EDGE ( 'NONE', *, *, #8990, .T. ) ;
#10510=DIRECTION ( 'NONE',  ( -0.000000000000000000, -0.000000000000000000, -1.000000000000000000 ) ) ;
#10513=ORIENTED_EDGE ( 'NONE', *, *, #6516, .F. ) ;
#10528=CARTESIAN_POINT ( 'NONE',  ( 29.49999999999999645, 2.000000000000001776, -5.500000000000000000 ) ) ;
#10547=DIRECTION ( 'NONE',  ( 1.248995262339999580E-16, -0.7071067811865463515, -0.7071067811865487940 ) ) ;
#10552=VECTOR ( 'NONE', #10359, 1000.000000000000000 ) ;
#10557=EDGE_CURVE ( 'NONE', #9304, #10287, #1019, .T. ) ;
#10563=VECTOR ( 'NONE', #3870, 1000.000000000000000 ) ;
#10567=AXIS2_PLACEMENT_3D ( 'NONE', #1721, #3881, #2947 ) ;
#10571=CIRCLE ( 'NONE', #9679, 4.500000000000000000 ) ;
#10580=DIRECTION ( 'NONE',  ( -1.000000000000000000, 9.251858538542971828E-16, 0.000000000000000000 ) ) ;
#10586=( NAMED_UNIT ( * ) SI_UNIT ( $, .STERADIAN. ) SOLID_ANGLE_UNIT ( ) );
#10603=SHAPE_REPRESENTATION ( 'caliper arm right', ( #308 ), #5109 ) ;
#10605=ORIENTED_EDGE ( 'NONE', *, *, #2900, .F. ) ;
#10617=AXIS2_PLACEMENT_3D ( 'NONE', #8051, #1438, #8208 ) ;
#10627=AXIS2_PLACEMENT_3D ( 'NONE', #10638, #7341, #2243 ) ;
#10631=CARTESIAN_POINT ( 'NONE',  ( -25.98076211353324894, 14.99999999999984190, -2.500000000000000000 ) ) ;
#10638=CARTESIAN_POINT ( 'NONE',  ( -25.71106610644865498, 0.000000000000000000, -5.000000000000000000 ) ) ;
#10645=ORIENTED_EDGE ( 'NONE', *, *, #9498, .F. ) ;
#10653=DIRECTION ( 'NONE',  ( -1.000000000000000000, 0.000000000000000000, 0.000000000000000000 ) ) ;
#10664=CARTESIAN_POINT ( 'NONE',  ( 34.66939513580730647, 4.803384628401708767, 2.499999999999999556 ) ) ;
#10665=ORIENTED_EDGE ( 'NONE', *, *, #236, .T. ) ;
#10676=DIRECTION ( 'NONE',  ( -1.000000000000000000, -0.000000000000000000, -0.000000000000000000 ) ) ;
#10679=ORIENTED_EDGE ( 'NONE', *, *, #10301, .F. ) ;
#10687=CARTESIAN_POINT ( 'NONE',  ( 34.99999999999999289, 1.431146867680865853E-14, -12.49999999999999822 ) ) ;
#10721=VECTOR ( 'NONE', #3652, 1000.000000000000000 ) ;
#10736=LINE ( 'NONE', #4700, #7199 ) ;
#10739=ORIENTED_EDGE ( 'NONE', *, *, #6670, .F. ) ;
#10740=AXIS2_PLACEMENT_3D ( 'NONE', #8246, #1582, #3247 ) ;
#10752=AXIS2_PLACEMENT_3D ( 'NONE', #361, #9033, #7255 ) ;
#10766=CARTESIAN_POINT ( 'NONE',  ( 34.64101615137754209, 5.000000000000000888, 2.500000000000000000 ) ) ;
#10777=LINE ( 'NONE', #820, #6119 ) ;
#10796=DIRECTION ( 'NONE',  ( 0.000000000000000000, 0.000000000000000000, 1.000000000000000000 ) ) ;
#10797=ORIENTED_EDGE ( 'NONE', *, *, #429, .F. ) ;
#10805=FACE_OUTER_BOUND ( 'NONE', #10932, .T. ) ;
#10808=DIRECTION ( 'NONE',  ( -0.000000000000000000, -0.000000000000000000, -1.000000000000000000 ) ) ;
#10810=ORIENTED_EDGE ( 'NONE', *, *, #838, .T. ) ;
#10819=ORIENTED_EDGE ( 'NONE', *, *, #9822, .F. ) ;
#10821=CARTESIAN_POINT ( 'NONE',  ( 34.80692069235084318, 3.675807134350209004, 2.800930295893637734 ) ) ;
#10823=EDGE_LOOP ( 'NONE', ( #8507, #7810, #8795 ) ) ;
#10843=AXIS2_PLACEMENT_3D ( 'NONE', #8641, #8582, #3640 ) ;
#10846=DIRECTION ( 'NONE',  ( 1.000000000000000000, -0.000000000000000000, -0.000000000000000000 ) ) ;
#10849=DIRECTION ( 'NONE',  ( 0.000000000000000000, 1.000000000000000000, 0.000000000000000000 ) ) ;
#10852=ORIENTED_EDGE ( 'NONE', *, *, #6968, .T. ) ;
#10857=VECTOR ( 'NONE', #7992, 1000.000000000000000 ) ;
#10861=DIRECTION ( 'NONE',  ( 0.000000000000000000, 1.000000000000000000, 0.000000000000000000 ) ) ;
#10865=VECTOR ( 'NONE', #691, 1000.000000000000000 ) ;
#10884=EDGE_CURVE ( 'NONE', #4463, #4583, #1978, .T. ) ;
#10900=CARTESIAN_POINT ( 'NONE',  ( 34.99999999999999289, -7.999999999999996447, -12.49999999999999822 ) ) ;
#10902=DIRECTION ( 'NONE',  ( 4.891728712884731355E-16, -0.7071067811865489050, -0.7071067811865462405 ) ) ;
#10904=VERTEX_POINT ( 'NONE', #3748 ) ;
#10905=DIRECTION ( 'NONE',  ( -1.000000000000000000, 0.000000000000000000, 0.000000000000000000 ) ) ;
#10911=AXIS2_PLACEMENT_3D ( 'NONE', #7333, #5679, #9844 ) ;
#10912=CARTESIAN_POINT ( 'NONE',  ( 34.76713615931383572, 4.034733667027951221, -2.652855901285303908 ) ) ;
#10914=CIRCLE ( 'NONE', #780, 34.99999999999999289 ) ;
#10918=EDGE_CURVE ( 'NONE', #4777, #8327, #8286, .T. ) ;
#10922=AXIS2_PLACEMENT_3D ( 'NONE', #1701, #5752, #8479 ) ;
#10930=ORIENTED_EDGE ( 'NONE', *, *, #3987, .T. ) ;
#10931=PLANE ( 'NONE',  #7583 ) ;
#10932=EDGE_LOOP ( 'NONE', ( #1544, #7681, #10259, #1210 ) ) ;
#10944=FACE_OUTER_BOUND ( 'NONE', #4346, .T. ) ;
#10947=FACE_OUTER_BOUND ( 'NONE', #8066, .T. ) ;
#10949=CARTESIAN_POINT ( 'NONE',  ( 34.99999999999999289, -17.99999999999998579, 7.500000000000053291 ) ) ;
#10955=ADVANCED_FACE ( 'NONE', ( #6357 ), #1075, .T. ) ;
#10972=DIRECTION ( 'NONE',  ( 0.000000000000000000, 0.000000000000000000, 1.000000000000000000 ) ) ;
#10974=AXIS2_PLACEMENT_3D ( 'NONE', #9416, #3310, #2656 ) ;
#10994=FACE_OUTER_BOUND ( 'NONE', #2374, .T. ) ;
ENDSEC;
END-ISO-10303-21;
